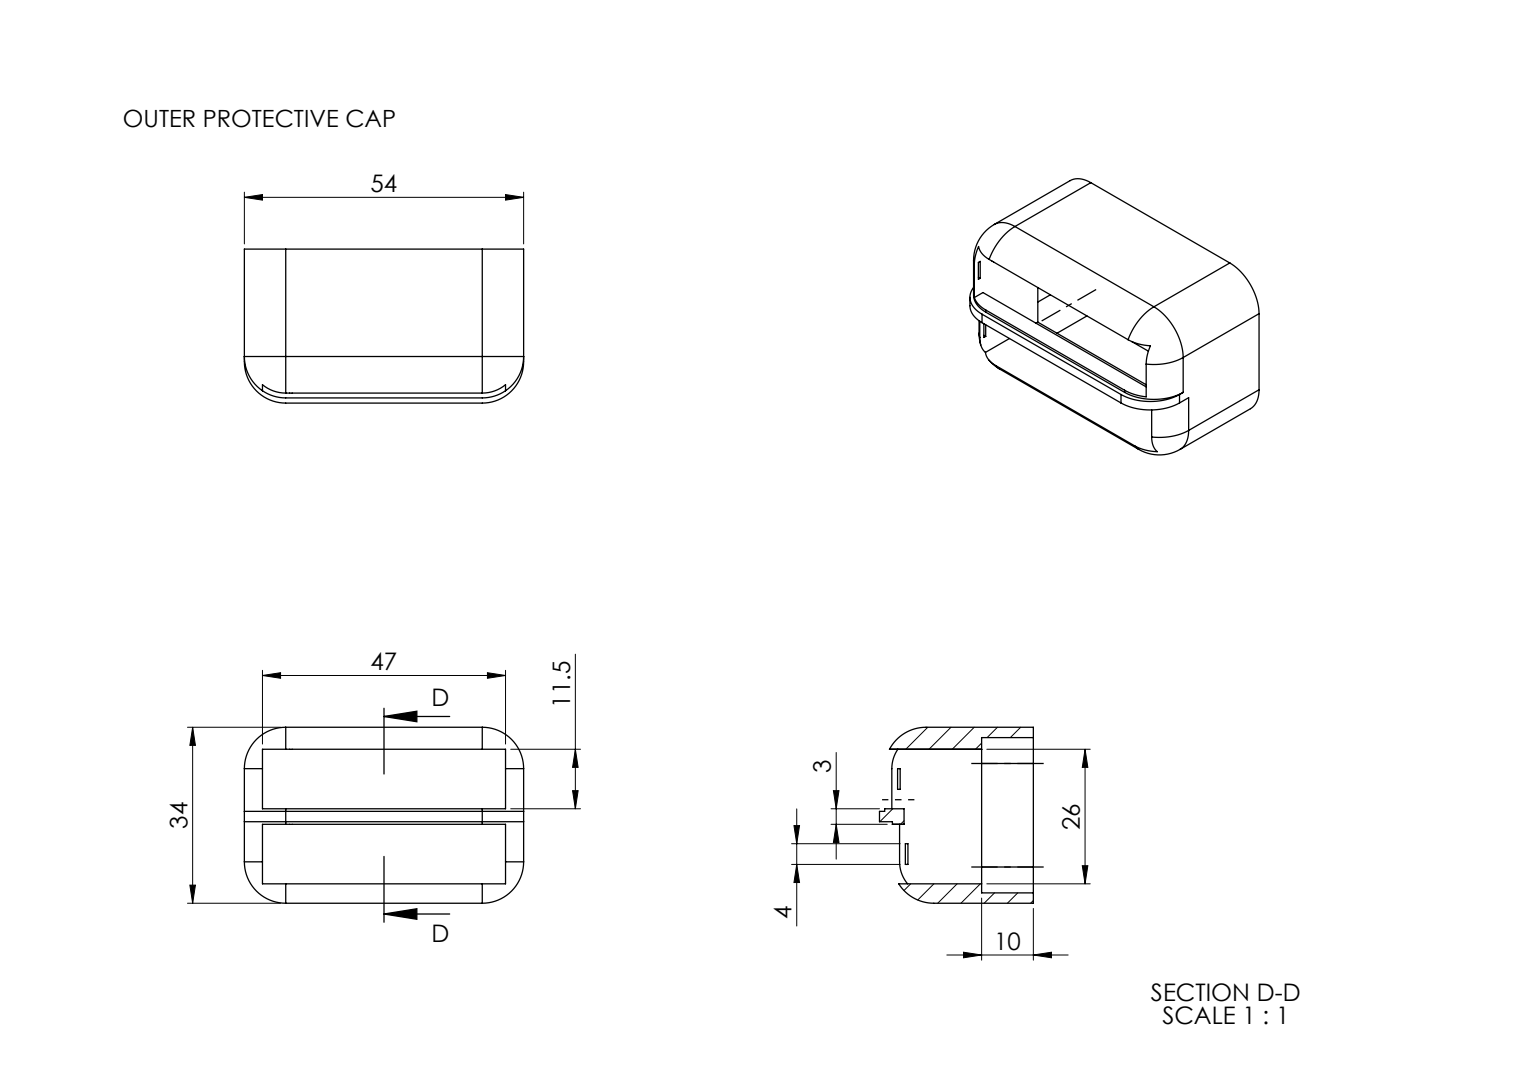
ISO-10303-21;
HEADER;
FILE_DESCRIPTION (('STEP AP214'),
    '1' );
FILE_NAME ('Outer Protective Cap.step',
    '2026-10-05T05:16:24',
    ( '' ),
    ( '' ),
    'SwSTEP 2.0',
    'SolidWorks 2026',
    '' );
FILE_SCHEMA (( 'AUTOMOTIVE_DESIGN' ));
ENDSEC;

DATA;
#39=VERTEX_POINT ( 'NONE', #74855 ) ;
#111=EDGE_LOOP ( 'NONE', ( #30455, #63884, #82521, #35885, #30536 ) ) ;
#125=ORIENTED_EDGE ( 'NONE', *, *, #59924, .F. ) ;
#176=DIRECTION ( 'NONE',  ( -1.000000000000000000, 1.799314243699348838E-16, 0.000000000000000000 ) ) ;
#177=VERTEX_POINT ( 'NONE', #56344 ) ;
#218=CYLINDRICAL_SURFACE ( 'NONE', #17781, 4.999999999999997335 ) ;
#355=CARTESIAN_POINT ( 'NONE',  ( -19.00000000000000355, 12.75000000000000888, 23.75000000000000000 ) ) ;
#369=EDGE_CURVE ( 'NONE', #87698, #17125, #35522, .T. ) ;
#423=VERTEX_POINT ( 'NONE', #22006 ) ;
#439=ORIENTED_EDGE ( 'NONE', *, *, #3601, .F. ) ;
#451=ORIENTED_EDGE ( 'NONE', *, *, #81392, .T. ) ;
#483=DIRECTION ( 'NONE',  ( -1.845450506358306311E-16, 1.000000000000000000, -5.102127870520021228E-17 ) ) ;
#523=VECTOR ( 'NONE', #26290, 1000.000000000000000 ) ;
#545=VERTEX_POINT ( 'NONE', #25105 ) ;
#584=DIRECTION ( 'NONE',  ( -1.000000000000000000, -0.000000000000000000, 0.000000000000000000 ) ) ;
#617=AXIS2_PLACEMENT_3D ( 'NONE', #45736, #44381, #25020 ) ;
#659=ORIENTED_EDGE ( 'NONE', *, *, #57921, .F. ) ;
#717=ADVANCED_FACE ( 'NONE', ( #61106 ), #88613, .F. ) ;
#728=DIRECTION ( 'NONE',  ( -1.000000000000000000, -0.000000000000000000, -0.000000000000000000 ) ) ;
#753=ORIENTED_EDGE ( 'NONE', *, *, #12775, .F. ) ;
#801=DIRECTION ( 'NONE',  ( -0.000000000000000000, -0.000000000000000000, -1.000000000000000000 ) ) ;
#834=DIRECTION ( 'NONE',  ( 0.000000000000000000, -1.000000000000000000, -0.000000000000000000 ) ) ;
#841=LINE ( 'NONE', #21553, #59983 ) ;
#876=ORIENTED_EDGE ( 'NONE', *, *, #18715, .F. ) ;
#913=CARTESIAN_POINT ( 'NONE',  ( 19.99999999999997513, -14.99999999999999467, 3.000000000000000888 ) ) ;
#976=CARTESIAN_POINT ( 'NONE',  ( -24.00000000000000000, 5.000000000000023093, 29.24999999999999645 ) ) ;
#1023=CIRCLE ( 'NONE', #35556, 4.755951259987792668 ) ;
#1024=DIRECTION ( 'NONE',  ( -0.000000000000000000, -0.000000000000000000, -1.000000000000000000 ) ) ;
#1050=CARTESIAN_POINT ( 'NONE',  ( 23.49999999999999645, 1.250000000000003775, 28.00000000000000000 ) ) ;
#1086=EDGE_CURVE ( 'NONE', #31481, #54731, #6721, .T. ) ;
#1098=DIRECTION ( 'NONE',  ( 0.000000000000000000, -1.084202172485503448E-16, 1.000000000000000000 ) ) ;
#1117=ORIENTED_EDGE ( 'NONE', *, *, #87020, .T. ) ;
#1198=CARTESIAN_POINT ( 'NONE',  ( 23.49999999999998934, 12.75000000000000711, 13.00000000000000178 ) ) ;
#1213=EDGE_LOOP ( 'NONE', ( #27297, #63065, #59456, #32063, #63736, #10968 ) ) ;
#1230=CARTESIAN_POINT ( 'NONE',  ( 20.00000000000000711, -9.999999999999994671, 13.00000000000000178 ) ) ;
#1264=DIRECTION ( 'NONE',  ( 0.000000000000000000, 8.131516293641283255E-17, 1.000000000000000000 ) ) ;
#1305=DIRECTION ( 'NONE',  ( 0.000000000000000000, -1.835858764360062270E-15, -1.000000000000000000 ) ) ;
#1341=EDGE_CURVE ( 'NONE', #39, #63016, #10830, .T. ) ;
#1369=VERTEX_POINT ( 'NONE', #40966 ) ;
#1370=DIRECTION ( 'NONE',  ( -8.673617379884044347E-16, 1.000000000000000000, -5.102127870520020612E-17 ) ) ;
#1444=CARTESIAN_POINT ( 'NONE',  ( 19.00000000000000000, 1.250000000000002220, 23.75000000000000000 ) ) ;
#1480=CARTESIAN_POINT ( 'NONE',  ( -17.76215049426127024, 12.75000000000001599, 30.81664701255127881 ) ) ;
#1523=DIRECTION ( 'NONE',  ( -1.000000000000000000, 5.997714145664496128E-17, -5.202187765341190574E-33 ) ) ;
#1557=LINE ( 'NONE', #29045, #38017 ) ;
#1675=VERTEX_POINT ( 'NONE', #16580 ) ;
#1704=FACE_OUTER_BOUND ( 'NONE', #66995, .T. ) ;
#2006=EDGE_CURVE ( 'NONE', #35616, #13977, #81696, .T. ) ;
#2165=CARTESIAN_POINT ( 'NONE',  ( 24.00000000000000000, 9.000000000000024869, 28.74999999999999645 ) ) ;
#2179=FILL_AREA_STYLE ('',( #15712 ) ) ;
#2260=ORIENTED_EDGE ( 'NONE', *, *, #66486, .F. ) ;
#2280=DIRECTION ( 'NONE',  ( -0.000000000000000000, -5.102127870520021228E-17, -1.000000000000000000 ) ) ;
#2292=CARTESIAN_POINT ( 'NONE',  ( 27.00000000000000000, 1.250000000000004663, 31.75000000000000000 ) ) ;
#2302=CARTESIAN_POINT ( 'NONE',  ( 19.00000000000000000, 17.00000000000000000, 2.999999999999999112 ) ) ;
#2374=CARTESIAN_POINT ( 'NONE',  ( -19.99999999999996803, 15.00000000000000711, 3.000000000000000000 ) ) ;
#2474=EDGE_CURVE ( 'NONE', #45845, #16480, #75885, .T. ) ;
#2476=CIRCLE ( 'NONE', #28394, 7.066647012551277918 ) ;
#2479=VERTEX_POINT ( 'NONE', #79605 ) ;
#2506=EDGE_LOOP ( 'NONE', ( #86542, #44118, #22143, #15946, #48903, #37980, #41332, #20143 ) ) ;
#2517=CARTESIAN_POINT ( 'NONE',  ( 27.00000000000000355, -1.749999999999999778, 30.25000000000000000 ) ) ;
#2532=ORIENTED_EDGE ( 'NONE', *, *, #18031, .T. ) ;
#2573=EDGE_CURVE ( 'NONE', #6905, #67687, #74625, .T. ) ;
#2625=CARTESIAN_POINT ( 'NONE',  ( -19.99999999999996447, -15.00000000000000533, 3.000000000000000000 ) ) ;
#2630=CIRCLE ( 'NONE', #81807, 4.999999999999997335 ) ;
#2700=ORIENTED_EDGE ( 'NONE', *, *, #82394, .F. ) ;
#2732=DIRECTION ( 'NONE',  ( -1.000000000000000000, 5.997714145664496128E-17, 0.000000000000000000 ) ) ;
#2785=ORIENTED_EDGE ( 'NONE', *, *, #6461, .T. ) ;
#2797=CARTESIAN_POINT ( 'NONE',  ( -19.99999999999996803, 15.00000000000000711, 13.00000000000000178 ) ) ;
#2836=LINE ( 'NONE', #37071, #56430 ) ;
#2885=VERTEX_POINT ( 'NONE', #13586 ) ;
#2953=VECTOR ( 'NONE', #7163, 1000.000000000000000 ) ;
#3016=CIRCLE ( 'NONE', #41878, 8.000000000000000000 ) ;
#3057=VERTEX_POINT ( 'NONE', #58111 ) ;
#3136=FACE_OUTER_BOUND ( 'NONE', #20499, .T. ) ;
#3200=ORIENTED_EDGE ( 'NONE', *, *, #34878, .F. ) ;
#3233=CARTESIAN_POINT ( 'NONE',  ( -23.50000000000000000, 9.000000000000024869, 28.74999999999999645 ) ) ;
#3297=SPHERICAL_SURFACE ( 'NONE', #10520, 8.000000000000000000 ) ;
#3359=CARTESIAN_POINT ( 'NONE',  ( 27.00000000000000000, 8.999999999999996447, 23.75000000000000000 ) ) ;
#3372=LINE ( 'NONE', #72275, #49878 ) ;
#3387=DIRECTION ( 'NONE',  ( 0.000000000000000000, -2.546383084002652634E-16, -1.000000000000000000 ) ) ;
#3399=ORIENTED_EDGE ( 'NONE', *, *, #32573, .T. ) ;
#3419=COLOUR_RGB ( '', 0.09019608, 0.27058824, 0.51372549) ;
#3420=VECTOR ( 'NONE', #31207, 1000.000000000000000 ) ;
#3466=EDGE_LOOP ( 'NONE', ( #67477, #25046, #38237, #39668, #79080, #56446 ) ) ;
#3504=( NAMED_UNIT ( * ) SI_UNIT ( $, .STERADIAN. ) SOLID_ANGLE_UNIT ( ) );
#3518=EDGE_CURVE ( 'NONE', #44526, #16365, #12061, .T. ) ;
#3601=EDGE_CURVE ( 'NONE', #21923, #31481, #62869, .T. ) ;
#3614=VECTOR ( 'NONE', #80699, 1000.000000000000000 ) ;
#3635=ORIENTED_EDGE ( 'NONE', *, *, #64166, .F. ) ;
#3658=ORIENTED_EDGE ( 'NONE', *, *, #34878, .T. ) ;
#3688=VERTEX_POINT ( 'NONE', #56578 ) ;
#3726=VERTEX_POINT ( 'NONE', #29556 ) ;
#3740=PLANE ( 'NONE',  #67370 ) ;
#3752=EDGE_LOOP ( 'NONE', ( #12490, #71544, #35024, #451, #52192 ) ) ;
#3764=VECTOR ( 'NONE', #64961, 1000.000000000000000 ) ;
#3860=DIRECTION ( 'NONE',  ( 0.000000000000000000, -8.673617379884028076E-17, -1.000000000000000000 ) ) ;
#3878=ORIENTED_EDGE ( 'NONE', *, *, #69519, .F. ) ;
#3888=FACE_OUTER_BOUND ( 'NONE', #46997, .T. ) ;
#3928=VECTOR ( 'NONE', #10062, 1000.000000000000000 ) ;
#3948=ORIENTED_EDGE ( 'NONE', *, *, #34547, .F. ) ;
#3952=VECTOR ( 'NONE', #74260, 1000.000000000000000 ) ;
#3976=ORIENTED_EDGE ( 'NONE', *, *, #4874, .T. ) ;
#4003=CARTESIAN_POINT ( 'NONE',  ( 19.99999999999996803, 15.00000000000000711, 3.000000000000000000 ) ) ;
#4012=AXIS2_PLACEMENT_3D ( 'NONE', #47900, #19109, #88476 ) ;
#4025=CARTESIAN_POINT ( 'NONE',  ( -24.00000000000000000, 5.000000000000023093, 28.74999999999999645 ) ) ;
#4098=CARTESIAN_POINT ( 'NONE',  ( 19.00000000000000000, -13.24999999999999822, 22.25000000000000000 ) ) ;
#4128=EDGE_CURVE ( 'NONE', #31550, #87883, #51453, .T. ) ;
#4149=VERTEX_POINT ( 'NONE', #66670 ) ;
#4163=DIRECTION ( 'NONE',  ( -1.000000000000000000, -1.734723475976813504E-16, 0.000000000000000000 ) ) ;
#4170=CARTESIAN_POINT ( 'NONE',  ( 23.49999999999998934, -9.499999999999982236, 32.75000000000000000 ) ) ;
#4179=DIRECTION ( 'NONE',  ( 0.000000000000000000, 0.000000000000000000, -1.000000000000000000 ) ) ;
#4246=FACE_OUTER_BOUND ( 'NONE', #51472, .T. ) ;
#4272=CARTESIAN_POINT ( 'NONE',  ( 19.00000000000000000, -9.000000000000001776, 3.000000000000000444 ) ) ;
#4339=VECTOR ( 'NONE', #88764, 1000.000000000000000 ) ;
#4430=VERTEX_POINT ( 'NONE', #52588 ) ;
#4613=AXIS2_PLACEMENT_3D ( 'NONE', #74305, #4163, #7172 ) ;
#4720=EDGE_CURVE ( 'NONE', #43004, #66583, #25016, .T. ) ;
#4766=AXIS2_PLACEMENT_3D ( 'NONE', #70291, #8598, #63525 ) ;
#4874=EDGE_CURVE ( 'NONE', #11165, #85470, #9196, .T. ) ;
#4886=EDGE_LOOP ( 'NONE', ( #16594, #13139, #67745, #50693, #20912, #63814, #12403, #82588, #60363, #32892 ) ) ;
#4972=CARTESIAN_POINT ( 'NONE',  ( 19.00000000000000000, 0.7500000000000051070, 32.75000000000000000 ) ) ;
#4981=VECTOR ( 'NONE', #68913, 1000.000000000000000 ) ;
#4993=DIRECTION ( 'NONE',  ( 0.000000000000000000, 0.000000000000000000, -1.000000000000000000 ) ) ;
#5019=DIRECTION ( 'NONE',  ( 0.000000000000000000, 0.000000000000000000, 1.000000000000000000 ) ) ;
#5041=VECTOR ( 'NONE', #66159, 1000.000000000000000 ) ;
#5227=PLANE ( 'NONE',  #65899 ) ;
#5246=CARTESIAN_POINT ( 'NONE',  ( -20.00000000000000355, -10.00000000000000533, 3.000000000000000000 ) ) ;
#5314=ORIENTED_EDGE ( 'NONE', *, *, #30408, .T. ) ;
#5316=EDGE_CURVE ( 'NONE', #76174, #11728, #59705, .T. ) ;
#5331=AXIS2_PLACEMENT_3D ( 'NONE', #20450, #41165, #176 ) ;
#5342=ADVANCED_FACE ( 'NONE', ( #24133 ), #71881, .F. ) ;
#5357=DIRECTION ( 'NONE',  ( -1.000000000000000000, 0.000000000000000000, 0.000000000000000000 ) ) ;
#5363=( NAMED_UNIT ( * ) SI_UNIT ( $, .STERADIAN. ) SOLID_ANGLE_UNIT ( ) );
#5367=ORIENTED_EDGE ( 'NONE', *, *, #53165, .F. ) ;
#5421=CARTESIAN_POINT ( 'NONE',  ( 24.00000000000000000, -5.499999999999981348, 27.75000000000000000 ) ) ;
#5486=EDGE_CURVE ( 'NONE', #30238, #88839, #84428, .T. ) ;
#5604=ORIENTED_EDGE ( 'NONE', *, *, #60963, .T. ) ;
#5642=VERTEX_POINT ( 'NONE', #24030 ) ;
#5646=VERTEX_POINT ( 'NONE', #59598 ) ;
#5699=ORIENTED_EDGE ( 'NONE', *, *, #76759, .F. ) ;
#5731=CARTESIAN_POINT ( 'NONE',  ( -23.50000000000000000, -4.999999999999999112, 28.00000000000000000 ) ) ;
#5735=CARTESIAN_POINT ( 'NONE',  ( 19.00000000000000000, -8.999999999999996447, 22.25000000000000000 ) ) ;
#5821=CARTESIAN_POINT ( 'NONE',  ( 23.49999999999998934, 1.674711738930281374E-15, 32.75000000000000000 ) ) ;
#5872=DIRECTION ( 'NONE',  ( 0.000000000000000000, 1.000000000000000000, 0.000000000000000000 ) ) ;
#5905=CYLINDRICAL_SURFACE ( 'NONE', #8415, 8.000000000000000000 ) ;
#5934=AXIS2_PLACEMENT_3D ( 'NONE', #51338, #37863, #45051 ) ;
#5952=LINE ( 'NONE', #26658, #24339 ) ;
#6010=VERTEX_POINT ( 'NONE', #26600 ) ;
#6014=CARTESIAN_POINT ( 'NONE',  ( 27.00000000000000000, -1.249999999999999112, 32.75000000000000000 ) ) ;
#6025=CARTESIAN_POINT ( 'NONE',  ( -24.00000000000000000, 9.000000000000024869, 29.25000000000000000 ) ) ;
#6048=CARTESIAN_POINT ( 'NONE',  ( 27.00000000000000000, -9.000000000000001776, 2.291744775602387568E-15 ) ) ;
#6069=CIRCLE ( 'NONE', #42074, 8.000000000000000000 ) ;
#6212=VECTOR ( 'NONE', #16061, 1000.000000000000000 ) ;
#6245=VECTOR ( 'NONE', #1098, 1000.000000000000000 ) ;
#6323=ADVANCED_FACE ( 'NONE', ( #53961 ), #81453, .T. ) ;
#6341=VECTOR ( 'NONE', #57691, 1000.000000000000000 ) ;
#6419=DIRECTION ( 'NONE',  ( -1.000000000000000000, 0.000000000000000000, 0.000000000000000000 ) ) ;
#6428=EDGE_CURVE ( 'NONE', #1675, #87698, #55728, .T. ) ;
#6459=ORIENTED_EDGE ( 'NONE', *, *, #78541, .F. ) ;
#6461=EDGE_CURVE ( 'NONE', #24326, #60483, #18351, .T. ) ;
#6465=ORIENTED_EDGE ( 'NONE', *, *, #8401, .F. ) ;
#6483=CYLINDRICAL_SURFACE ( 'NONE', #4012, 4.755951259987790891 ) ;
#6495=PLANE ( 'NONE',  #5331 ) ;
#6503=CIRCLE ( 'NONE', #79853, 8.000000000000000000 ) ;
#6589=ORIENTED_EDGE ( 'NONE', *, *, #17057, .F. ) ;
#6714=LINE ( 'NONE', #48575, #2953 ) ;
#6721=CIRCLE ( 'NONE', #57038, 7.066647012551277918 ) ;
#6795=ADVANCED_FACE ( 'NONE', ( #39027, #31822 ), #5227, .F. ) ;
#6808=DIRECTION ( 'NONE',  ( -1.000000000000000000, 0.000000000000000000, 0.000000000000000000 ) ) ;
#6905=VERTEX_POINT ( 'NONE', #78005 ) ;
#6909=ORIENTED_EDGE ( 'NONE', *, *, #29491, .T. ) ;
#6949=EDGE_LOOP ( 'NONE', ( #61040, #37601, #63641, #78757, #20835, #88190, #51917, #53034, #28989, #28438 ) ) ;
#6996=VECTOR ( 'NONE', #75423, 1000.000000000000000 ) ;
#7127=CARTESIAN_POINT ( 'NONE',  ( -19.99999999999996803, 15.00000000000000711, 13.00000000000000178 ) ) ;
#7136=DIRECTION ( 'NONE',  ( 0.000000000000000000, 1.000000000000000000, 8.673617379884033500E-16 ) ) ;
#7163=DIRECTION ( 'NONE',  ( -0.000000000000000000, -5.102127870520021228E-17, -1.000000000000000000 ) ) ;
#7172=DIRECTION ( 'NONE',  ( 1.734723475976813504E-16, -1.000000000000000000, 0.000000000000000000 ) ) ;
#7189=LINE ( 'NONE', #27018, #85069 ) ;
#7271=DIRECTION ( 'NONE',  ( 0.000000000000000000, 0.000000000000000000, 1.000000000000000000 ) ) ;
#7286=EDGE_LOOP ( 'NONE', ( #59348, #15601, #28024, #83746 ) ) ;
#7302=VECTOR ( 'NONE', #32279, 1000.000000000000000 ) ;
#7321=EDGE_CURVE ( 'NONE', #76030, #46479, #65704, .T. ) ;
#7424=PRODUCT ( 'Outer Protective Cap', 'Outer Protective Cap', '', ( #53651 ) ) ;
#7435=EDGE_CURVE ( 'NONE', #79431, #62505, #2630, .T. ) ;
#7437=EDGE_LOOP ( 'NONE', ( #68832, #81407, #41481, #25142 ) ) ;
#7496=CARTESIAN_POINT ( 'NONE',  ( -23.50000000000000000, 12.75000000000000533, 32.75000000000000000 ) ) ;
#7508=PLANE ( 'NONE',  #35416 ) ;
#7555=DIRECTION ( 'NONE',  ( -1.000000000000000000, -9.819216796286635314E-16, -2.454804199071659026E-15 ) ) ;
#7556=DIRECTION ( 'NONE',  ( 1.000000000000000000, 0.000000000000000000, 0.000000000000000000 ) ) ;
#7579=PRESENTATION_STYLE_ASSIGNMENT (( #34156 ) ) ;
#7587=CARTESIAN_POINT ( 'NONE',  ( -24.00000000000000000, -9.499999999999982236, 27.74999999999999645 ) ) ;
#7626=VERTEX_POINT ( 'NONE', #72360 ) ;
#7648=CARTESIAN_POINT ( 'NONE',  ( -24.00000000000000000, 9.000000000000024869, 28.74999999999999645 ) ) ;
#7726=CARTESIAN_POINT ( 'NONE',  ( 23.49999999999998934, -9.499999999999982236, 27.24999999999999645 ) ) ;
#7740=EDGE_LOOP ( 'NONE', ( #55686, #47275, #8190, #46826, #38658, #51031, #61137, #86767 ) ) ;
#7762=DIRECTION ( 'NONE',  ( 5.997714145664496128E-17, 1.000000000000000000, -5.102127870520021228E-17 ) ) ;
#7817=VERTEX_POINT ( 'NONE', #53418 ) ;
#7988=DIRECTION ( 'NONE',  ( -1.000000000000000000, 1.681660752236433198E-16, 0.000000000000000000 ) ) ;
#8011=DIRECTION ( 'NONE',  ( 0.000000000000000000, -1.000000000000000000, 0.000000000000000000 ) ) ;
#8013=VERTEX_POINT ( 'NONE', #57860 ) ;
#8034=CARTESIAN_POINT ( 'NONE',  ( -19.00000000000000000, -1.249999999999997558, 22.25000000000000000 ) ) ;
#8098=ORIENTED_EDGE ( 'NONE', *, *, #38884, .T. ) ;
#8113=ORIENTED_EDGE ( 'NONE', *, *, #2474, .T. ) ;
#8128=LINE ( 'NONE', #8570, #54588 ) ;
#8138=PLANE ( 'NONE',  #17965 ) ;
#8140=CARTESIAN_POINT ( 'NONE',  ( -17.76215049426128445, -1.749999999999992450, 28.00000000000000000 ) ) ;
#8190=ORIENTED_EDGE ( 'NONE', *, *, #7435, .F. ) ;
#8196=CARTESIAN_POINT ( 'NONE',  ( 23.49999999999999645, -4.999999999999999112, 28.00000000000000000 ) ) ;
#8219=VERTEX_POINT ( 'NONE', #1050 ) ;
#8232=DIRECTION ( 'NONE',  ( 0.000000000000000000, 0.000000000000000000, -1.000000000000000000 ) ) ;
#8240=CARTESIAN_POINT ( 'NONE',  ( 24.00000000000000000, 5.000000000000023093, 29.24999999999999645 ) ) ;
#8260=VECTOR ( 'NONE', #9877, 1000.000000000000000 ) ;
#8266=ORIENTED_EDGE ( 'NONE', *, *, #26687, .F. ) ;
#8267=VECTOR ( 'NONE', #45746, 1000.000000000000000 ) ;
#8384=DIRECTION ( 'NONE',  ( 0.000000000000000000, 0.000000000000000000, -1.000000000000000000 ) ) ;
#8401=EDGE_CURVE ( 'NONE', #11121, #17125, #86987, .T. ) ;
#8415=AXIS2_PLACEMENT_3D ( 'NONE', #33381, #60839, #33813 ) ;
#8570=CARTESIAN_POINT ( 'NONE',  ( 23.49999999999998579, -13.25000000000000000, 32.75000000000000000 ) ) ;
#8590=DIRECTION ( 'NONE',  ( -1.000000000000000000, 0.000000000000000000, -0.000000000000000000 ) ) ;
#8598=DIRECTION ( 'NONE',  ( 0.000000000000000000, -5.102127870520020612E-17, -1.000000000000000000 ) ) ;
#8626=LINE ( 'NONE', #36535, #16851 ) ;
#8636=LINE ( 'NONE', #2292, #13220 ) ;
#8670=DIRECTION ( 'NONE',  ( 0.000000000000000000, 1.084202172485504434E-16, -1.000000000000000000 ) ) ;
#8720=DIRECTION ( 'NONE',  ( -0.000000000000000000, 1.000000000000000000, 0.000000000000000000 ) ) ;
#8746=ADVANCED_FACE ( 'NONE', ( #30164 ), #49552, .F. ) ;
#8750=EDGE_CURVE ( 'NONE', #87698, #26806, #49101, .T. ) ;
#8767=DIRECTION ( 'NONE',  ( 0.000000000000000000, -1.000000000000000000, 0.000000000000000000 ) ) ;
#8791=DIRECTION ( 'NONE',  ( -0.000000000000000000, -1.000000000000000000, -8.673617379884033500E-16 ) ) ;
#8793=AXIS2_PLACEMENT_3D ( 'NONE', #28742, #56206, #42260 ) ;
#8833=CARTESIAN_POINT ( 'NONE',  ( -27.00000000000000000, 0.7500000000000059952, 24.75000000000000000 ) ) ;
#8844=EDGE_CURVE ( 'NONE', #79547, #52311, #8128, .T. ) ;
#8863=ORIENTED_EDGE ( 'NONE', *, *, #8401, .T. ) ;
#8892=ORIENTED_EDGE ( 'NONE', *, *, #22887, .F. ) ;
#9065=EDGE_LOOP ( 'NONE', ( #69141, #36454, #49626, #49654 ) ) ;
#9076=AXIS2_PLACEMENT_3D ( 'NONE', #58222, #44698, #23116 ) ;
#9108=ORIENTED_EDGE ( 'NONE', *, *, #84957, .T. ) ;
#9143=ORIENTED_EDGE ( 'NONE', *, *, #25495, .T. ) ;
#9196=LINE ( 'NONE', #71314, #3928 ) ;
#9238=CARTESIAN_POINT ( 'NONE',  ( -24.00000000000000000, 9.000000000000024869, 29.25000000000000000 ) ) ;
#9245=ADVANCED_FACE ( 'NONE', ( #4246 ), #32605, .F. ) ;
#9328=EDGE_LOOP ( 'NONE', ( #60045, #3948, #71017, #78144 ) ) ;
#9390=ORIENTED_EDGE ( 'NONE', *, *, #12535, .F. ) ;
#9391=LINE ( 'NONE', #44479, #86633 ) ;
#9442=DIRECTION ( 'NONE',  ( -0.000000000000000000, -0.000000000000000000, -1.000000000000000000 ) ) ;
#9446=DIRECTION ( 'NONE',  ( 0.000000000000000000, 0.000000000000000000, 1.000000000000000000 ) ) ;
#9454=EDGE_CURVE ( 'NONE', #81222, #85470, #45970, .T. ) ;
#9506=ORIENTED_EDGE ( 'NONE', *, *, #18954, .T. ) ;
#9638=ORIENTED_EDGE ( 'NONE', *, *, #38910, .T. ) ;
#9679=EDGE_CURVE ( 'NONE', #76954, #66225, #76195, .T. ) ;
#9687=ORIENTED_EDGE ( 'NONE', *, *, #70774, .F. ) ;
#9877=DIRECTION ( 'NONE',  ( -0.000000000000000000, -0.000000000000000000, -1.000000000000000000 ) ) ;
#9880=DIRECTION ( 'NONE',  ( 1.000000000000000000, -0.000000000000000000, -0.000000000000000000 ) ) ;
#9914=ORIENTED_EDGE ( 'NONE', *, *, #12070, .F. ) ;
#9922=VERTEX_POINT ( 'NONE', #15788 ) ;
#9924=FACE_OUTER_BOUND ( 'NONE', #12091, .T. ) ;
#10003=ORIENTED_EDGE ( 'NONE', *, *, #60963, .F. ) ;
#10009=LINE ( 'NONE', #2797, #85627 ) ;
#10062=DIRECTION ( 'NONE',  ( -0.000000000000000000, 1.000000000000000000, -0.000000000000000000 ) ) ;
#10068=VECTOR ( 'NONE', #29097, 1000.000000000000000 ) ;
#10078=DIRECTION ( 'NONE',  ( -0.000000000000000000, 1.000000000000000000, -0.000000000000000000 ) ) ;
#10191=CARTESIAN_POINT ( 'NONE',  ( -24.00000000000000000, -5.499999999999981348, 27.75000000000000000 ) ) ;
#10198=AXIS2_PLACEMENT_3D ( 'NONE', #51631, #79136, #17437 ) ;
#10253=DIRECTION ( 'NONE',  ( 0.000000000000000000, -1.000000000000000000, -8.673617379884033500E-16 ) ) ;
#10353=CARTESIAN_POINT ( 'NONE',  ( 27.00000000000000000, -16.99999999999999289, 30.25000000000000000 ) ) ;
#10520=AXIS2_PLACEMENT_3D ( 'NONE', #59132, #37525, #64991 ) ;
#10602=CARTESIAN_POINT ( 'NONE',  ( 23.49999999999998934, 12.75000000000000888, 32.75000000000000000 ) ) ;
#10661=PLANE ( 'NONE',  #23127 ) ;
#10666=DIRECTION ( 'NONE',  ( 0.000000000000000000, 0.000000000000000000, -1.000000000000000000 ) ) ;
#10732=VECTOR ( 'NONE', #79377, 1000.000000000000000 ) ;
#10742=ORIENTED_EDGE ( 'NONE', *, *, #73680, .F. ) ;
#10782=LINE ( 'NONE', #30165, #5041 ) ;
#10819=PLANE ( 'NONE',  #74194 ) ;
#10830=LINE ( 'NONE', #80639, #41309 ) ;
#10912=LINE ( 'NONE', #70848, #72096 ) ;
#10943=ORIENTED_EDGE ( 'NONE', *, *, #30776, .F. ) ;
#10968=ORIENTED_EDGE ( 'NONE', *, *, #71445, .F. ) ;
#11027=DIRECTION ( 'NONE',  ( -0.000000000000000000, -5.102127870520021228E-17, -1.000000000000000000 ) ) ;
#11028=ORIENTED_EDGE ( 'NONE', *, *, #20816, .T. ) ;
#11082=EDGE_CURVE ( 'NONE', #65772, #45114, #6714, .T. ) ;
#11121=VERTEX_POINT ( 'NONE', #55339 ) ;
#11142=AXIS2_PLACEMENT_3D ( 'NONE', #10191, #52495, #66467 ) ;
#11165=VERTEX_POINT ( 'NONE', #60771 ) ;
#11270=CARTESIAN_POINT ( 'NONE',  ( 24.00000000000000000, 9.000000000000024869, 29.25000000000000000 ) ) ;
#11394=DIRECTION ( 'NONE',  ( -1.000000000000000000, 0.000000000000000000, 0.000000000000000000 ) ) ;
#11416=VECTOR ( 'NONE', #32266, 1000.000000000000000 ) ;
#11440=CARTESIAN_POINT ( 'NONE',  ( 23.49999999999998934, -9.499999999999982236, 27.74999999999999645 ) ) ;
#11472=LINE ( 'NONE', #79929, #40463 ) ;
#11479=CARTESIAN_POINT ( 'NONE',  ( -23.50000000000000000, 1.250000000000005329, 32.75000000000000000 ) ) ;
#11544=CARTESIAN_POINT ( 'NONE',  ( 27.00000000000000000, 17.00000000000000000, 2.999999999999999112 ) ) ;
#11580=DIRECTION ( 'NONE',  ( 1.000000000000000000, -0.000000000000000000, -0.000000000000000000 ) ) ;
#11610=DIRECTION ( 'NONE',  ( 0.000000000000000000, 1.000000000000000000, -8.673617379884035472E-17 ) ) ;
#11625=PRODUCT_DEFINITION_FORMATION_WITH_SPECIFIED_SOURCE ( 'ANY', '', #7424, .NOT_KNOWN. ) ;
#11661=DIRECTION ( 'NONE',  ( 0.000000000000000000, -1.000000000000000000, 4.336808689942017736E-16 ) ) ;
#11684=ORIENTED_EDGE ( 'NONE', *, *, #44990, .F. ) ;
#11728=VERTEX_POINT ( 'NONE', #55960 ) ;
#11777=ORIENTED_EDGE ( 'NONE', *, *, #68590, .T. ) ;
#11801=ORIENTED_EDGE ( 'NONE', *, *, #55924, .T. ) ;
#11815=DIRECTION ( 'NONE',  ( 0.000000000000000000, -1.734723475976807094E-15, 1.000000000000000000 ) ) ;
#11898=CARTESIAN_POINT ( 'NONE',  ( -24.00000000000000000, -5.499999999999981348, 27.25000000000000000 ) ) ;
#11968=EDGE_CURVE ( 'NONE', #58506, #69466, #3016, .T. ) ;
#12061=LINE ( 'NONE', #5731, #21237 ) ;
#12070=EDGE_CURVE ( 'NONE', #64945, #68629, #11472, .T. ) ;
#12091=EDGE_LOOP ( 'NONE', ( #9390, #73108, #41023, #25285 ) ) ;
#12093=EDGE_LOOP ( 'NONE', ( #35540, #62139, #69676, #3635 ) ) ;
#12118=CARTESIAN_POINT ( 'NONE',  ( 27.00000000000000000, 16.99999999999999289, 31.75000000000000000 ) ) ;
#12132=EDGE_LOOP ( 'NONE', ( #40428, #59501, #85620, #21590 ) ) ;
#12133=AXIS2_PLACEMENT_3D ( 'NONE', #47495, #34430, #34866 ) ;
#12180=CIRCLE ( 'NONE', #20789, 7.999999999999998224 ) ;
#12194=FACE_OUTER_BOUND ( 'NONE', #55388, .T. ) ;
#12341=AXIS2_PLACEMENT_3D ( 'NONE', #80947, #39070, #65182 ) ;
#12400=DIRECTION ( 'NONE',  ( -0.000000000000000000, -5.102127870520021228E-17, -1.000000000000000000 ) ) ;
#12403=ORIENTED_EDGE ( 'NONE', *, *, #79194, .F. ) ;
#12427=CARTESIAN_POINT ( 'NONE',  ( 19.00000000000000000, -17.00000000000000000, 2.999999999999999112 ) ) ;
#12478=AXIS2_PLACEMENT_3D ( 'NONE', #7587, #47680, #14337 ) ;
#12490=ORIENTED_EDGE ( 'NONE', *, *, #75862, .F. ) ;
#12528=ORIENTED_EDGE ( 'NONE', *, *, #57921, .T. ) ;
#12529=EDGE_CURVE ( 'NONE', #43877, #88176, #27980, .T. ) ;
#12535=EDGE_CURVE ( 'NONE', #31022, #56583, #72080, .T. ) ;
#12737=ORIENTED_EDGE ( 'NONE', *, *, #80670, .F. ) ;
#12775=EDGE_CURVE ( 'NONE', #13977, #73914, #87377, .T. ) ;
#12832=ORIENTED_EDGE ( 'NONE', *, *, #60564, .T. ) ;
#12961=EDGE_CURVE ( 'NONE', #47159, #43004, #52013, .T. ) ;
#13110=DIRECTION ( 'NONE',  ( 0.000000000000000000, 1.000000000000000000, 0.000000000000000000 ) ) ;
#13139=ORIENTED_EDGE ( 'NONE', *, *, #87746, .T. ) ;
#13141=DIRECTION ( 'NONE',  ( 1.000000000000000000, 0.000000000000000000, 0.000000000000000000 ) ) ;
#13181=ADVANCED_FACE ( 'NONE', ( #88945 ), #55126, .T. ) ;
#13220=VECTOR ( 'NONE', #2732, 1000.000000000000000 ) ;
#13419=CARTESIAN_POINT ( 'NONE',  ( -39.05038313613820122, 12.25000000000000711, 28.74999999999999645 ) ) ;
#13422=DIRECTION ( 'NONE',  ( 0.000000000000000000, -1.000000000000000000, 0.000000000000000000 ) ) ;
#13448=PLANE ( 'NONE',  #12478 ) ;
#13488=CARTESIAN_POINT ( 'NONE',  ( 27.00000000000000000, 0.7500000000000052180, 31.75000000000000000 ) ) ;
#13582=CARTESIAN_POINT ( 'NONE',  ( 23.49999999999998934, 4.710477821889702467E-15, 29.24999999999999289 ) ) ;
#13586=CARTESIAN_POINT ( 'NONE',  ( -19.00000000000000000, 17.00000000000000000, 2.999999999999999112 ) ) ;
#13646=AXIS2_PLACEMENT_3D ( 'NONE', #80003, #19958, #59280 ) ;
#13662=CARTESIAN_POINT ( 'NONE',  ( 25.00000000000000355, 9.999999999999971578, 13.00000000000000178 ) ) ;
#13714=CARTESIAN_POINT ( 'NONE',  ( 27.00000000000000000, 0.000000000000000000, 23.75000000000000000 ) ) ;
#13755=DIRECTION ( 'NONE',  ( 0.000000000000000000, 0.000000000000000000, 1.000000000000000000 ) ) ;
#13820=EDGE_CURVE ( 'NONE', #38892, #11165, #6069, .T. ) ;
#13855=DIRECTION ( 'NONE',  ( -1.000000000000000000, -0.000000000000000000, -0.000000000000000000 ) ) ;
#13869=ORIENTED_EDGE ( 'NONE', *, *, #52559, .F. ) ;
#13883=SURFACE_STYLE_FILL_AREA ( #48105 ) ;
#13920=AXIS2_PLACEMENT_3D ( 'NONE', #60216, #26885, #54343 ) ;
#13977=VERTEX_POINT ( 'NONE', #62544 ) ;
#14033=EDGE_CURVE ( 'NONE', #53401, #77030, #9391, .T. ) ;
#14162=VERTEX_POINT ( 'NONE', #79175 ) ;
#14170=CARTESIAN_POINT ( 'NONE',  ( -20.00000000000000355, -10.00000000000000533, 13.00000000000000178 ) ) ;
#14242=DIRECTION ( 'NONE',  ( 0.000000000000000000, -1.000000000000000000, 0.000000000000000000 ) ) ;
#14284=AXIS2_PLACEMENT_3D ( 'NONE', #71255, #72148, #36602 ) ;
#14294=FACE_OUTER_BOUND ( 'NONE', #9328, .T. ) ;
#14318=CARTESIAN_POINT ( 'NONE',  ( 27.00000000000000000, 0.7500000000000061062, 23.75000000000000000 ) ) ;
#14337=DIRECTION ( 'NONE',  ( 0.000000000000000000, 0.000000000000000000, -1.000000000000000000 ) ) ;
#14379=CIRCLE ( 'NONE', #50288, 4.999999999999997335 ) ;
#14394=ORIENTED_EDGE ( 'NONE', *, *, #79644, .F. ) ;
#14490=EDGE_CURVE ( 'NONE', #62484, #43877, #22349, .T. ) ;
#14577=UNCERTAINTY_MEASURE_WITH_UNIT (LENGTH_MEASURE( 1.000000000000000082E-05 ), #80064, 'distance_accuracy_value', 'NONE');
#14606=LINE ( 'NONE', #13714, #16418 ) ;
#14608=CARTESIAN_POINT ( 'NONE',  ( -25.00000000000000355, 9.999999999999971578, 3.000000000000000000 ) ) ;
#14613=CARTESIAN_POINT ( 'NONE',  ( -18.00000000000001421, 17.49999999999802824, 32.75000000000000000 ) ) ;
#14621=EDGE_LOOP ( 'NONE', ( #8892, #26121, #83182, #81793 ) ) ;
#14656=CARTESIAN_POINT ( 'NONE',  ( -27.00000000000000000, -1.250000000000000000, 22.25000000000000000 ) ) ;
#14706=ORIENTED_EDGE ( 'NONE', *, *, #53045, .F. ) ;
#14716=EDGE_LOOP ( 'NONE', ( #43267, #46097, #3399, #57529 ) ) ;
#14756=CARTESIAN_POINT ( 'NONE',  ( 23.49999999999998934, 5.000000000000023093, 28.74999999999999645 ) ) ;
#14820=ADVANCED_FACE ( 'NONE', ( #71636 ), #57689, .T. ) ;
#14842=AXIS2_PLACEMENT_3D ( 'NONE', #69439, #43300, #55914 ) ;
#14851=DIRECTION ( 'NONE',  ( 0.000000000000000000, -1.000000000000000000, 0.000000000000000000 ) ) ;
#14864=LINE ( 'NONE', #20285, #51703 ) ;
#14890=DIRECTION ( 'NONE',  ( 0.000000000000000000, 0.000000000000000000, -1.000000000000000000 ) ) ;
#14965=ORIENTED_EDGE ( 'NONE', *, *, #28232, .T. ) ;
#14969=ORIENTED_EDGE ( 'NONE', *, *, #56579, .T. ) ;
#15048=LINE ( 'NONE', #42523, #19719 ) ;
#15076=DIRECTION ( 'NONE',  ( 1.000000000000000000, -0.000000000000000000, -0.000000000000000000 ) ) ;
#15105=VECTOR ( 'NONE', #70409, 1000.000000000000000 ) ;
#15156=EDGE_CURVE ( 'NONE', #3726, #58506, #7189, .T. ) ;
#15215=CARTESIAN_POINT ( 'NONE',  ( 19.00000000000000000, 0.000000000000000000, 24.75000000000000000 ) ) ;
#15276=AXIS2_PLACEMENT_3D ( 'NONE', #75743, #6419, #82079 ) ;
#15312=ORIENTED_EDGE ( 'NONE', *, *, #29870, .T. ) ;
#15326=ADVANCED_FACE ( 'NONE', ( #29054 ), #22280, .F. ) ;
#15329=CARTESIAN_POINT ( 'NONE',  ( 24.00000000000000000, 14.50000000000000533, 1.499999999999997780 ) ) ;
#15542=DIRECTION ( 'NONE',  ( -1.799314243699348838E-16, -1.000000000000000000, 5.102127870520021228E-17 ) ) ;
#15585=DIRECTION ( 'NONE',  ( -0.000000000000000000, -5.102127870520021228E-17, -1.000000000000000000 ) ) ;
#15596=CARTESIAN_POINT ( 'NONE',  ( -24.00000000000000000, -9.499999999999982236, 27.74999999999999645 ) ) ;
#15601=ORIENTED_EDGE ( 'NONE', *, *, #84957, .F. ) ;
#15624=EDGE_CURVE ( 'NONE', #44546, #9922, #69323, .T. ) ;
#15654=CARTESIAN_POINT ( 'NONE',  ( 23.49999999999998579, -8.999999999999996447, 28.86437827766148345 ) ) ;
#15712=FILL_AREA_STYLE_COLOUR ( '', #3419 ) ;
#15771=CARTESIAN_POINT ( 'NONE',  ( 24.00000000000000000, 9.000000000000024869, 29.25000000000000000 ) ) ;
#15788=CARTESIAN_POINT ( 'NONE',  ( 27.00000000000000000, 0.7500000000000059952, 24.75000000000000000 ) ) ;
#15849=VERTEX_POINT ( 'NONE', #32928 ) ;
#15943=VERTEX_POINT ( 'NONE', #21176 ) ;
#15946=ORIENTED_EDGE ( 'NONE', *, *, #29149, .T. ) ;
#15976=VECTOR ( 'NONE', #53324, 1000.000000000000000 ) ;
#15985=EDGE_LOOP ( 'NONE', ( #23359, #38033, #42032, #3200 ) ) ;
#15989=LINE ( 'NONE', #9238, #57236 ) ;
#15999=DIRECTION ( 'NONE',  ( 0.000000000000000000, -1.000000000000000000, 4.336808689942017736E-16 ) ) ;
#16061=DIRECTION ( 'NONE',  ( -0.000000000000000000, -0.000000000000000000, -1.000000000000000000 ) ) ;
#16063=ORIENTED_EDGE ( 'NONE', *, *, #42110, .F. ) ;
#16102=CARTESIAN_POINT ( 'NONE',  ( 27.00000000000000000, 0.000000000000000000, 22.25000000000000000 ) ) ;
#16116=EDGE_CURVE ( 'NONE', #56516, #69466, #81019, .T. ) ;
#16138=EDGE_CURVE ( 'NONE', #88830, #56373, #73362, .T. ) ;
#16351=FACE_OUTER_BOUND ( 'NONE', #7286, .T. ) ;
#16365=VERTEX_POINT ( 'NONE', #33495 ) ;
#16418=VECTOR ( 'NONE', #41194, 1000.000000000000000 ) ;
#16427=EDGE_LOOP ( 'NONE', ( #45138, #48937, #69979, #35694 ) ) ;
#16450=ORIENTED_EDGE ( 'NONE', *, *, #50493, .F. ) ;
#16479=AXIS2_PLACEMENT_3D ( 'NONE', #63920, #86445, #37331 ) ;
#16480=VERTEX_POINT ( 'NONE', #83909 ) ;
#16500=DIRECTION ( 'NONE',  ( 0.000000000000000000, -1.000000000000000000, -8.673617379884033500E-16 ) ) ;
#16578=DIRECTION ( 'NONE',  ( 0.000000000000000000, 0.000000000000000000, -1.000000000000000000 ) ) ;
#16580=CARTESIAN_POINT ( 'NONE',  ( 24.00000000000000000, 5.000000000000023093, 28.74999999999999645 ) ) ;
#16594=ORIENTED_EDGE ( 'NONE', *, *, #64615, .T. ) ;
#16731=UNCERTAINTY_MEASURE_WITH_UNIT (LENGTH_MEASURE( 1.000000000000000082E-05 ), #73373, 'distance_accuracy_value', 'NONE');
#16758=CARTESIAN_POINT ( 'NONE',  ( 27.00000000000000000, 0.000000000000000000, 0.000000000000000000 ) ) ;
#16760=CIRCLE ( 'NONE', #52704, 8.000000000000000000 ) ;
#16794=CARTESIAN_POINT ( 'NONE',  ( 7.497142682080633102E-17, 1.250000000000003553, 28.00000000000000000 ) ) ;
#16823=VECTOR ( 'NONE', #23413, 1000.000000000000000 ) ;
#16851=VECTOR ( 'NONE', #2280, 1000.000000000000000 ) ;
#16906=CYLINDRICAL_SURFACE ( 'NONE', #27624, 8.000000000000000000 ) ;
#17055=ORIENTED_EDGE ( 'NONE', *, *, #66336, .T. ) ;
#17057=EDGE_CURVE ( 'NONE', #88830, #13977, #32839, .T. ) ;
#17061=DIRECTION ( 'NONE',  ( 0.000000000000000000, 1.000000000000000000, 8.673617379884034486E-16 ) ) ;
#17081=LINE ( 'NONE', #56739, #8260 ) ;
#17086=AXIS2_PLACEMENT_3D ( 'NONE', #12118, #83229, #54863 ) ;
#17125=VERTEX_POINT ( 'NONE', #33727 ) ;
#17131=EDGE_LOOP ( 'NONE', ( #9506, #70627, #17055, #68156, #39911, #67901, #63783, #41654 ) ) ;
#17294=DIRECTION ( 'NONE',  ( 0.000000000000000000, 0.000000000000000000, 1.000000000000000000 ) ) ;
#17389=VECTOR ( 'NONE', #9880, 1000.000000000000000 ) ;
#17416=LINE ( 'NONE', #80004, #85092 ) ;
#17417=EDGE_LOOP ( 'NONE', ( #2260, #85181, #55144, #53399 ) ) ;
#17437=DIRECTION ( 'NONE',  ( 1.000000000000000000, 0.000000000000000000, 0.000000000000000000 ) ) ;
#17511=LINE ( 'NONE', #51712, #25894 ) ;
#17521=FACE_OUTER_BOUND ( 'NONE', #80523, .T. ) ;
#17591=FACE_OUTER_BOUND ( 'NONE', #38414, .T. ) ;
#17614=ORIENTED_EDGE ( 'NONE', *, *, #33771, .F. ) ;
#17740=ORIENTED_EDGE ( 'NONE', *, *, #73680, .T. ) ;
#17781=AXIS2_PLACEMENT_3D ( 'NONE', #14170, #41646, #69115 ) ;
#17788=ORIENTED_EDGE ( 'NONE', *, *, #50706, .F. ) ;
#17817=DIRECTION ( 'NONE',  ( -0.000000000000000000, -5.102127870520021228E-17, -1.000000000000000000 ) ) ;
#17841=AXIS2_PLACEMENT_3D ( 'NONE', #75858, #75420, #68221 ) ;
#17878=DIRECTION ( 'NONE',  ( 0.000000000000000000, 0.000000000000000000, 1.000000000000000000 ) ) ;
#17925=ORIENTED_EDGE ( 'NONE', *, *, #31578, .F. ) ;
#17965=AXIS2_PLACEMENT_3D ( 'NONE', #83808, #1370, #42374 ) ;
#18018=CARTESIAN_POINT ( 'NONE',  ( 7.497142682080631869E-17, 1.250000000000003775, 32.75000000000000000 ) ) ;
#18031=EDGE_CURVE ( 'NONE', #7626, #2885, #82439, .T. ) ;
#18036=ORIENTED_EDGE ( 'NONE', *, *, #22131, .F. ) ;
#18109=DIRECTION ( 'NONE',  ( 0.000000000000000000, 0.000000000000000000, 1.000000000000000000 ) ) ;
#18122=ORIENTED_EDGE ( 'NONE', *, *, #14490, .T. ) ;
#18127=VECTOR ( 'NONE', #728, 1000.000000000000000 ) ;
#18154=ORIENTED_EDGE ( 'NONE', *, *, #88340, .F. ) ;
#18166=VERTEX_POINT ( 'NONE', #77763 ) ;
#18320=AXIS2_PLACEMENT_3D ( 'NONE', #31184, #34188, #19793 ) ;
#18351=CIRCLE ( 'NONE', #68676, 5.000000000000000888 ) ;
#18359=CARTESIAN_POINT ( 'NONE',  ( -23.50000000000000000, 1.674711738930281374E-15, 13.00000000000000178 ) ) ;
#18380=LINE ( 'NONE', #2625, #49219 ) ;
#18519=CARTESIAN_POINT ( 'NONE',  ( -24.00000000000000000, -9.499999999999982236, 27.74999999999999645 ) ) ;
#18582=EDGE_LOOP ( 'NONE', ( #69344, #44033, #11028, #60832 ) ) ;
#18597=EDGE_CURVE ( 'NONE', #4430, #44526, #27348, .T. ) ;
#18623=CARTESIAN_POINT ( 'NONE',  ( 24.00000000000000000, -5.499999999999981348, 27.25000000000000000 ) ) ;
#18680=EDGE_CURVE ( 'NONE', #52311, #4149, #64658, .T. ) ;
#18715=EDGE_CURVE ( 'NONE', #19020, #34521, #79969, .T. ) ;
#18750=DIRECTION ( 'NONE',  ( -1.000000000000000000, 0.000000000000000000, 0.000000000000000000 ) ) ;
#18755=ORIENTED_EDGE ( 'NONE', *, *, #66486, .T. ) ;
#18863=CARTESIAN_POINT ( 'NONE',  ( 27.00000000000000000, -17.00000000000000000, 2.999999999999999112 ) ) ;
#18905=ADVANCED_FACE ( 'NONE', ( #69114 ), #33994, .T. ) ;
#18953=CARTESIAN_POINT ( 'NONE',  ( 24.00000000000000000, -9.499999999999982236, 27.25000000000000000 ) ) ;
#18954=EDGE_CURVE ( 'NONE', #45845, #9922, #34439, .T. ) ;
#19020=VERTEX_POINT ( 'NONE', #29909 ) ;
#19051=DIRECTION ( 'NONE',  ( 0.000000000000000000, 0.000000000000000000, 1.000000000000000000 ) ) ;
#19098=EDGE_CURVE ( 'NONE', #5646, #2479, #65452, .T. ) ;
#19109=DIRECTION ( 'NONE',  ( -0.000000000000000000, -5.102127870520021228E-17, -1.000000000000000000 ) ) ;
#19122=ORIENTED_EDGE ( 'NONE', *, *, #1086, .F. ) ;
#19125=DIRECTION ( 'NONE',  ( -0.000000000000000000, -5.102127870520021228E-17, -1.000000000000000000 ) ) ;
#19144=ADVANCED_FACE ( 'NONE', ( #79425, #44726 ), #32556, .F. ) ;
#19191=VECTOR ( 'NONE', #17061, 1000.000000000000000 ) ;
#19266=CYLINDRICAL_SURFACE ( 'NONE', #45755, 8.000000000000000000 ) ;
#19307=DIRECTION ( 'NONE',  ( 0.000000000000000000, 1.000000000000000000, 5.102127870520020612E-17 ) ) ;
#19315=AXIS2_PLACEMENT_3D ( 'NONE', #55062, #67255, #27590 ) ;
#19336=FACE_BOUND ( 'NONE', #83331, .T. ) ;
#19352=ORIENTED_EDGE ( 'NONE', *, *, #85635, .F. ) ;
#19360=CARTESIAN_POINT ( 'NONE',  ( -19.00000000000000000, 0.7500000000000041078, 23.75000000000000000 ) ) ;
#19391=DIRECTION ( 'NONE',  ( 1.000000000000000000, 0.000000000000000000, 0.000000000000000000 ) ) ;
#19393=CARTESIAN_POINT ( 'NONE',  ( -24.00000000000000000, -5.499999999999981348, 27.75000000000000000 ) ) ;
#19564=DIRECTION ( 'NONE',  ( 0.000000000000000000, -5.102127870520020612E-17, -1.000000000000000000 ) ) ;
#19625=ADVANCED_FACE ( 'NONE', ( #49518 ), #22043, .T. ) ;
#19643=CARTESIAN_POINT ( 'NONE',  ( -27.00000000000000000, 8.999999999999996447, 23.75000000000000000 ) ) ;
#19703=CARTESIAN_POINT ( 'NONE',  ( -19.00000000000000000, 0.7500000000000051070, 24.75000000000000000 ) ) ;
#19719=VECTOR ( 'NONE', #48819, 1000.000000000000000 ) ;
#19737=DIRECTION ( 'NONE',  ( 1.000000000000000000, 0.000000000000000000, 0.000000000000000000 ) ) ;
#19769=VECTOR ( 'NONE', #76730, 1000.000000000000000 ) ;
#19779=FACE_OUTER_BOUND ( 'NONE', #62503, .T. ) ;
#19793=DIRECTION ( 'NONE',  ( 0.000000000000000000, -1.000000000000000000, 8.673617379884035472E-17 ) ) ;
#19828=LINE ( 'NONE', #43198, #24840 ) ;
#19912=AXIS2_PLACEMENT_3D ( 'NONE', #40103, #68878, #55364 ) ;
#19940=DIRECTION ( 'NONE',  ( 0.000000000000000000, 2.413528314402514090E-16, -1.000000000000000000 ) ) ;
#19958=DIRECTION ( 'NONE',  ( -0.000000000000000000, -0.000000000000000000, -1.000000000000000000 ) ) ;
#19990=AXIS2_PLACEMENT_3D ( 'NONE', #15215, #8011, #49438 ) ;
#20043=CARTESIAN_POINT ( 'NONE',  ( -23.50000000000000000, -13.25000000000000888, 32.75000000000000000 ) ) ;
#20115=VECTOR ( 'NONE', #33356, 1000.000000000000000 ) ;
#20132=DIRECTION ( 'NONE',  ( 0.000000000000000000, 2.413528314402514090E-16, -1.000000000000000000 ) ) ;
#20143=ORIENTED_EDGE ( 'NONE', *, *, #57350, .T. ) ;
#20199=DIRECTION ( 'NONE',  ( 0.000000000000000000, -4.336808689942017736E-16, 1.000000000000000000 ) ) ;
#20226=CARTESIAN_POINT ( 'NONE',  ( 19.00000000000000000, 8.999999999999996447, 23.75000000000000000 ) ) ;
#20285=CARTESIAN_POINT ( 'NONE',  ( 24.00000000000000000, 5.000000000000023093, 28.74999999999999645 ) ) ;
#20286=ORIENTED_EDGE ( 'NONE', *, *, #26687, .T. ) ;
#20374=CARTESIAN_POINT ( 'NONE',  ( 25.00000000000000711, -9.999999999999957367, 3.000000000000000000 ) ) ;
#20436=FACE_OUTER_BOUND ( 'NONE', #17417, .T. ) ;
#20450=CARTESIAN_POINT ( 'NONE',  ( -3.148799926473854982E-16, -1.749999999999995559, 32.75000000000000000 ) ) ;
#20499=EDGE_LOOP ( 'NONE', ( #32129, #9638, #52720, #46190, #72294, #21600 ) ) ;
#20789=AXIS2_PLACEMENT_3D ( 'NONE', #87333, #26502, #80572 ) ;
#20816=EDGE_CURVE ( 'NONE', #44546, #61438, #41787, .T. ) ;
#20835=ORIENTED_EDGE ( 'NONE', *, *, #80670, .T. ) ;
#20849=DIRECTION ( 'NONE',  ( -1.000000000000000000, 0.000000000000000000, 0.000000000000000000 ) ) ;
#20867=ORIENTED_EDGE ( 'NONE', *, *, #34345, .F. ) ;
#20879=ORIENTED_EDGE ( 'NONE', *, *, #13820, .T. ) ;
#20909=DIRECTION ( 'NONE',  ( -0.000000000000000000, -1.000000000000000000, 8.673617379884028076E-17 ) ) ;
#20912=ORIENTED_EDGE ( 'NONE', *, *, #41392, .T. ) ;
#20970=DIRECTION ( 'NONE',  ( 0.000000000000000000, -5.102127870520020612E-17, -1.000000000000000000 ) ) ;
#21017=DIRECTION ( 'NONE',  ( -0.000000000000000000, -5.102127870520021228E-17, -1.000000000000000000 ) ) ;
#21024=ORIENTED_EDGE ( 'NONE', *, *, #78582, .F. ) ;
#21087=EDGE_CURVE ( 'NONE', #6010, #15849, #25239, .T. ) ;
#21115=FACE_OUTER_BOUND ( 'NONE', #87965, .T. ) ;
#21176=CARTESIAN_POINT ( 'NONE',  ( -19.00000000000000000, -1.249999999999999334, 30.25000000000000000 ) ) ;
#21237=VECTOR ( 'NONE', #11610, 1000.000000000000000 ) ;
#21363=CARTESIAN_POINT ( 'NONE',  ( -19.00000000000000355, 12.75000000000004974, 30.81664701255125394 ) ) ;
#21405=DIRECTION ( 'NONE',  ( -0.000000000000000000, -0.000000000000000000, 1.000000000000000000 ) ) ;
#21406=ADVANCED_FACE ( 'NONE', ( #40649 ), #48274, .F. ) ;
#21437=EDGE_CURVE ( 'NONE', #66225, #79431, #63561, .T. ) ;
#21475=CARTESIAN_POINT ( 'NONE',  ( -27.00000000000000000, 9.000000000000001776, 2.999999999999995559 ) ) ;
#21514=AXIS2_PLACEMENT_3D ( 'NONE', #46039, #66310, #23538 ) ;
#21533=ORIENTED_EDGE ( 'NONE', *, *, #30408, .F. ) ;
#21553=CARTESIAN_POINT ( 'NONE',  ( -23.50000000000000000, 4.710477821889702467E-15, 29.24999999999999289 ) ) ;
#21590=ORIENTED_EDGE ( 'NONE', *, *, #31636, .F. ) ;
#21591=DIRECTION ( 'NONE',  ( -2.602085213965214586E-16, 1.000000000000000000, 0.000000000000000000 ) ) ;
#21600=ORIENTED_EDGE ( 'NONE', *, *, #63620, .T. ) ;
#21649=COLOUR_RGB ( '', 0.09019608, 0.27058824, 0.51372549) ;
#21691=ADVANCED_FACE ( 'NONE', ( #69695 ), #68811, .T. ) ;
#21739=FACE_OUTER_BOUND ( 'NONE', #46081, .T. ) ;
#21786=DIRECTION ( 'NONE',  ( 0.000000000000000000, -0.000000000000000000, -1.000000000000000000 ) ) ;
#21806=ORIENTED_EDGE ( 'NONE', *, *, #34547, .T. ) ;
#21830=ORIENTED_EDGE ( 'NONE', *, *, #59924, .T. ) ;
#21917=EDGE_CURVE ( 'NONE', #11165, #64684, #86338, .T. ) ;
#21923=VERTEX_POINT ( 'NONE', #73246 ) ;
#21952=EDGE_CURVE ( 'NONE', #57828, #87883, #45940, .T. ) ;
#22006=CARTESIAN_POINT ( 'NONE',  ( -23.50000000000000000, 9.000000000000024869, 29.25000000000000000 ) ) ;
#22029=EDGE_CURVE ( 'NONE', #79431, #33821, #35705, .T. ) ;
#22040=DIRECTION ( 'NONE',  ( -1.000000000000000000, -2.602085213965214586E-16, 0.000000000000000000 ) ) ;
#22043=CYLINDRICAL_SURFACE ( 'NONE', #85607, 8.000000000000000000 ) ;
#22131=EDGE_CURVE ( 'NONE', #63016, #67027, #31596, .T. ) ;
#22143=ORIENTED_EDGE ( 'NONE', *, *, #19098, .T. ) ;
#22203=CARTESIAN_POINT ( 'NONE',  ( -23.50000000000000000, 1.250000000000005329, 30.36437827766147279 ) ) ;
#22214=APPLICATION_CONTEXT ( 'automotive_design' ) ;
#22224=ADVANCED_FACE ( 'NONE', ( #23067 ), #53645, .T. ) ;
#22247=CARTESIAN_POINT ( 'NONE',  ( 25.00000000000000711, -9.999999999999957367, 13.00000000000000178 ) ) ;
#22280=PLANE ( 'NONE',  #24685 ) ;
#22349=LINE ( 'NONE', #15596, #64861 ) ;
#22477=DIRECTION ( 'NONE',  ( 0.000000000000000000, 0.000000000000000000, 1.000000000000000000 ) ) ;
#22538=ORIENTED_EDGE ( 'NONE', *, *, #71445, .T. ) ;
#22646=EDGE_CURVE ( 'NONE', #79547, #65630, #22914, .T. ) ;
#22724=EDGE_LOOP ( 'NONE', ( #37684, #23079, #19352, #16063 ) ) ;
#22732=CIRCLE ( 'NONE', #19912, 5.000000000000000888 ) ;
#22802=DIRECTION ( 'NONE',  ( -1.000000000000000000, -0.000000000000000000, -0.000000000000000000 ) ) ;
#22808=CARTESIAN_POINT ( 'NONE',  ( 25.00000000000000355, 9.999999999999971578, 13.00000000000000178 ) ) ;
#22850=DIRECTION ( 'NONE',  ( 0.000000000000000000, -1.000000000000000000, 0.000000000000000000 ) ) ;
#22887=EDGE_CURVE ( 'NONE', #33821, #78112, #14379, .T. ) ;
#22914=CIRCLE ( 'NONE', #86206, 6.614378277661484340 ) ;
#22915=CIRCLE ( 'NONE', #34436, 8.000000000000000000 ) ;
#23067=FACE_OUTER_BOUND ( 'NONE', #64989, .T. ) ;
#23079=ORIENTED_EDGE ( 'NONE', *, *, #27744, .F. ) ;
#23105=DIRECTION ( 'NONE',  ( -0.000000000000000000, -5.102127870520021228E-17, -1.000000000000000000 ) ) ;
#23113=CARTESIAN_POINT ( 'NONE',  ( -19.00000000000000000, -16.99999999999999645, 22.25000000000000355 ) ) ;
#23116=DIRECTION ( 'NONE',  ( 0.000000000000000000, 0.000000000000000000, -1.000000000000000000 ) ) ;
#23127=AXIS2_PLACEMENT_3D ( 'NONE', #31374, #24611, #59733 ) ;
#23144=ORIENTED_EDGE ( 'NONE', *, *, #21087, .F. ) ;
#23161=CARTESIAN_POINT ( 'NONE',  ( -24.00000000000000000, 9.000000000000024869, 29.25000000000000000 ) ) ;
#23354=VECTOR ( 'NONE', #23683, 1000.000000000000000 ) ;
#23359=ORIENTED_EDGE ( 'NONE', *, *, #34020, .T. ) ;
#23390=VERTEX_POINT ( 'NONE', #33949 ) ;
#23393=DIRECTION ( 'NONE',  ( -0.000000000000000000, -0.000000000000000000, 1.000000000000000000 ) ) ;
#23413=DIRECTION ( 'NONE',  ( 1.000000000000000000, -0.000000000000000000, -0.000000000000000000 ) ) ;
#23480=AXIS2_PLACEMENT_3D ( 'NONE', #54605, #19940, #87547 ) ;
#23538=DIRECTION ( 'NONE',  ( 0.000000000000000000, 1.084202172485504434E-16, -1.000000000000000000 ) ) ;
#23588=CARTESIAN_POINT ( 'NONE',  ( -23.50000000000000000, -9.499999999999982236, 27.74999999999999645 ) ) ;
#23609=CIRCLE ( 'NONE', #17841, 8.000000000000000000 ) ;
#23612=ORIENTED_EDGE ( 'NONE', *, *, #6428, .T. ) ;
#23676=CARTESIAN_POINT ( 'NONE',  ( 27.00000000000000000, -16.99999999999999645, 22.25000000000000355 ) ) ;
#23683=DIRECTION ( 'NONE',  ( 1.000000000000000000, -1.799314243699348838E-16, 0.000000000000000000 ) ) ;
#23773=EDGE_CURVE ( 'NONE', #67027, #15943, #67678, .T. ) ;
#23990=DIRECTION ( 'NONE',  ( 0.000000000000000000, 0.000000000000000000, 1.000000000000000000 ) ) ;
#24030=CARTESIAN_POINT ( 'NONE',  ( 19.99999999999996803, 15.00000000000000711, 13.00000000000000178 ) ) ;
#24133=FACE_OUTER_BOUND ( 'NONE', #25365, .T. ) ;
#24179=PLANE ( 'NONE',  #10198 ) ;
#24233=DIRECTION ( 'NONE',  ( -0.000000000000000000, -1.000000000000000000, 8.673617379884035472E-17 ) ) ;
#24274=EDGE_CURVE ( 'NONE', #56516, #76174, #66244, .T. ) ;
#24295=DIRECTION ( 'NONE',  ( -0.000000000000000000, 0.000000000000000000, -1.000000000000000000 ) ) ;
#24326=VERTEX_POINT ( 'NONE', #79499 ) ;
#24327=LINE ( 'NONE', #72525, #74342 ) ;
#24339=VECTOR ( 'NONE', #60884, 1000.000000000000000 ) ;
#24393=DIRECTION ( 'NONE',  ( -0.000000000000000000, -0.000000000000000000, -1.000000000000000000 ) ) ;
#24486=CARTESIAN_POINT ( 'NONE',  ( -25.00000000000000355, 9.999999999999971578, 13.00000000000000178 ) ) ;
#24496=DIRECTION ( 'NONE',  ( 0.000000000000000000, 0.000000000000000000, -1.000000000000000000 ) ) ;
#24611=DIRECTION ( 'NONE',  ( 1.000000000000000000, 1.734723475976812518E-16, -0.000000000000000000 ) ) ;
#24638=CARTESIAN_POINT ( 'NONE',  ( -24.00000000000000000, -5.499999999999981348, 27.75000000000000000 ) ) ;
#24663=LINE ( 'NONE', #18359, #28212 ) ;
#24685=AXIS2_PLACEMENT_3D ( 'NONE', #23161, #25385, #17294 ) ;
#24751=DIRECTION ( 'NONE',  ( 1.000000000000000000, 0.000000000000000000, -0.000000000000000000 ) ) ;
#24840=VECTOR ( 'NONE', #28347, 1000.000000000000000 ) ;
#24909=CARTESIAN_POINT ( 'NONE',  ( 27.00000000000000000, -1.249999999999999112, 32.75000000000000000 ) ) ;
#24955=ORIENTED_EDGE ( 'NONE', *, *, #2006, .F. ) ;
#24998=ORIENTED_EDGE ( 'NONE', *, *, #76662, .T. ) ;
#25016=LINE ( 'NONE', #45733, #86056 ) ;
#25020=DIRECTION ( 'NONE',  ( 1.000000000000000000, 0.000000000000000000, 0.000000000000000000 ) ) ;
#25030=STYLED_ITEM ( 'NONE', ( #71522 ), #29637 ) ;
#25046=ORIENTED_EDGE ( 'NONE', *, *, #74844, .F. ) ;
#25054=CARTESIAN_POINT ( 'NONE',  ( 27.00000000000000000, -8.999999999999996447, 22.25000000000000000 ) ) ;
#25105=CARTESIAN_POINT ( 'NONE',  ( -23.50000000000000000, 12.75000000000000355, 29.19862367942583603 ) ) ;
#25142=ORIENTED_EDGE ( 'NONE', *, *, #8750, .F. ) ;
#25224=VERTEX_POINT ( 'NONE', #33902 ) ;
#25239=CIRCLE ( 'NONE', #75566, 8.000000000000000000 ) ;
#25272=SPHERICAL_SURFACE ( 'NONE', #48040, 8.000000000000000000 ) ;
#25285=ORIENTED_EDGE ( 'NONE', *, *, #38205, .T. ) ;
#25324=EDGE_LOOP ( 'NONE', ( #47375, #6465, #52543, #36998 ) ) ;
#25365=EDGE_LOOP ( 'NONE', ( #41088, #41114, #80654, #40729 ) ) ;
#25380=ORIENTED_EDGE ( 'NONE', *, *, #369, .T. ) ;
#25381=ORIENTED_EDGE ( 'NONE', *, *, #85984, .T. ) ;
#25385=DIRECTION ( 'NONE',  ( 0.000000000000000000, 1.000000000000000000, -0.000000000000000000 ) ) ;
#25435=DIRECTION ( 'NONE',  ( 0.000000000000000000, 1.000000000000000000, 0.000000000000000000 ) ) ;
#25495=EDGE_CURVE ( 'NONE', #87883, #79547, #75006, .T. ) ;
#25496=DIRECTION ( 'NONE',  ( -0.000000000000000000, -1.000000000000000000, -0.000000000000000000 ) ) ;
#25499=DIRECTION ( 'NONE',  ( -0.000000000000000000, 5.102127870520020612E-17, 1.000000000000000000 ) ) ;
#25545=DIRECTION ( 'NONE',  ( 0.000000000000000000, -1.000000000000000000, -1.084202172485503448E-16 ) ) ;
#25546=ORIENTED_EDGE ( 'NONE', *, *, #1341, .T. ) ;
#25574=FACE_OUTER_BOUND ( 'NONE', #29296, .T. ) ;
#25629=( NAMED_UNIT ( * ) PLANE_ANGLE_UNIT ( ) SI_UNIT ( $, .RADIAN. ) );
#25686=CARTESIAN_POINT ( 'NONE',  ( -24.00000000000000000, 9.000000000000024869, 28.74999999999999645 ) ) ;
#25705=DIRECTION ( 'NONE',  ( 0.000000000000000000, 0.000000000000000000, -1.000000000000000000 ) ) ;
#25785=ADVANCED_FACE ( 'NONE', ( #58051 ), #37784, .T. ) ;
#25802=AXIS2_PLACEMENT_3D ( 'NONE', #26296, #53765, #26739 ) ;
#25859=ORIENTED_EDGE ( 'NONE', *, *, #11082, .T. ) ;
#25894=VECTOR ( 'NONE', #30569, 1000.000000000000000 ) ;
#25949=MECHANICAL_DESIGN_GEOMETRIC_PRESENTATION_REPRESENTATION('',(#79192),#40366);
#25952=DIRECTION ( 'NONE',  ( 1.000000000000000000, -0.000000000000000000, -0.000000000000000000 ) ) ;
#25970=CARTESIAN_POINT ( 'NONE',  ( -19.99999999999996447, -15.00000000000000533, 13.00000000000000178 ) ) ;
#26009=CIRCLE ( 'NONE', #37504, 8.000000000000000000 ) ;
#26020=DIRECTION ( 'NONE',  ( -1.000000000000000000, 0.000000000000000000, 0.000000000000000000 ) ) ;
#26121=ORIENTED_EDGE ( 'NONE', *, *, #22029, .F. ) ;
#26151=LINE ( 'NONE', #19393, #41647 ) ;
#26174=EDGE_CURVE ( 'NONE', #44526, #68629, #17416, .T. ) ;
#26176=CARTESIAN_POINT ( 'NONE',  ( -19.00000000000000000, -16.99999999999999289, 22.25000000000000000 ) ) ;
#26187=PLANE ( 'NONE',  #51913 ) ;
#26197=EDGE_LOOP ( 'NONE', ( #63824, #49549, #72030, #26483 ) ) ;
#26248=DIRECTION ( 'NONE',  ( 0.000000000000000000, -1.000000000000000000, -8.673617379884033500E-16 ) ) ;
#26268=VECTOR ( 'NONE', #45277, 1000.000000000000000 ) ;
#26290=DIRECTION ( 'NONE',  ( -1.734723475976813750E-16, 1.000000000000000000, -0.000000000000000000 ) ) ;
#26296=CARTESIAN_POINT ( 'NONE',  ( 27.00000000000000000, 0.7500000000000052180, 31.75000000000000000 ) ) ;
#26297=VECTOR ( 'NONE', #15585, 1000.000000000000000 ) ;
#26395=EDGE_CURVE ( 'NONE', #54784, #31550, #44829, .T. ) ;
#26403=CARTESIAN_POINT ( 'NONE',  ( -23.50000000000000000, 8.999999999999996447, 23.75000000000000000 ) ) ;
#26407=CARTESIAN_POINT ( 'NONE',  ( -23.50000000000000000, -16.99999999999999289, 28.86437827766147279 ) ) ;
#26409=ADVANCED_FACE ( 'NONE', ( #76342 ), #84010, .F. ) ;
#26483=ORIENTED_EDGE ( 'NONE', *, *, #21952, .T. ) ;
#26502=DIRECTION ( 'NONE',  ( -0.000000000000000000, -4.336808689942017243E-16, -1.000000000000000000 ) ) ;
#26600=CARTESIAN_POINT ( 'NONE',  ( 27.00000000000000000, 8.999999999999996447, 23.75000000000000000 ) ) ;
#26658=CARTESIAN_POINT ( 'NONE',  ( 24.00000000000000000, 5.000000000000023093, 29.24999999999999645 ) ) ;
#26683=ORIENTED_EDGE ( 'NONE', *, *, #48219, .F. ) ;
#26687=EDGE_CURVE ( 'NONE', #54790, #18166, #53752, .T. ) ;
#26701=CYLINDRICAL_SURFACE ( 'NONE', #23480, 8.000000000000000000 ) ;
#26739=DIRECTION ( 'NONE',  ( 0.000000000000000000, 1.084202172485503448E-16, -1.000000000000000000 ) ) ;
#26800=LINE ( 'NONE', #20043, #49400 ) ;
#26806=VERTEX_POINT ( 'NONE', #78339 ) ;
#26829=ORIENTED_EDGE ( 'NONE', *, *, #15624, .T. ) ;
#26885=DIRECTION ( 'NONE',  ( 1.845450506358306311E-16, -1.000000000000000000, 5.102127870520020612E-17 ) ) ;
#26930=CARTESIAN_POINT ( 'NONE',  ( -39.05038313613820122, -2.249999999999999556, 27.25000000000000000 ) ) ;
#26936=ORIENTED_EDGE ( 'NONE', *, *, #80257, .T. ) ;
#27018=CARTESIAN_POINT ( 'NONE',  ( 19.00000000000000000, 16.99999999999999289, 31.75000000000000000 ) ) ;
#27092=DIRECTION ( 'NONE',  ( 1.000000000000000000, -0.000000000000000000, -0.000000000000000000 ) ) ;
#27138=EDGE_CURVE ( 'NONE', #55802, #79573, #28741, .T. ) ;
#27158=DIRECTION ( 'NONE',  ( 0.000000000000000000, -8.673617379884028076E-17, -1.000000000000000000 ) ) ;
#27180=VECTOR ( 'NONE', #5872, 1000.000000000000000 ) ;
#27297=ORIENTED_EDGE ( 'NONE', *, *, #41392, .F. ) ;
#27306=LINE ( 'NONE', #44230, #15105 ) ;
#27348=LINE ( 'NONE', #35427, #37867 ) ;
#27590=DIRECTION ( 'NONE',  ( 0.000000000000000000, 2.546383084002652634E-16, 1.000000000000000000 ) ) ;
#27612=VECTOR ( 'NONE', #22850, 1000.000000000000000 ) ;
#27624=AXIS2_PLACEMENT_3D ( 'NONE', #65079, #3387, #38068 ) ;
#27737=CARTESIAN_POINT ( 'NONE',  ( 19.00000000000000000, 9.000000000000001776, 2.999999999999999556 ) ) ;
#27744=EDGE_CURVE ( 'NONE', #79573, #56516, #60535, .T. ) ;
#27812=LINE ( 'NONE', #48970, #47493 ) ;
#27820=CARTESIAN_POINT ( 'NONE',  ( 24.00000000000000000, 9.000000000000024869, 28.74999999999999645 ) ) ;
#27923=ORIENTED_EDGE ( 'NONE', *, *, #369, .F. ) ;
#27957=ORIENTED_EDGE ( 'NONE', *, *, #4128, .T. ) ;
#27967=CARTESIAN_POINT ( 'NONE',  ( -1.105886215935217678E-14, 12.75000000000002487, 13.00000000000000178 ) ) ;
#27980=LINE ( 'NONE', #68963, #60572 ) ;
#28024=ORIENTED_EDGE ( 'NONE', *, *, #88503, .T. ) ;
#28155=ORIENTED_EDGE ( 'NONE', *, *, #32573, .F. ) ;
#28190=CARTESIAN_POINT ( 'NONE',  ( 23.49999999999998934, 1.674711738930281374E-15, 13.00000000000000178 ) ) ;
#28212=VECTOR ( 'NONE', #52127, 1000.000000000000000 ) ;
#28232=EDGE_CURVE ( 'NONE', #76954, #31022, #48092, .T. ) ;
#28347=DIRECTION ( 'NONE',  ( -0.000000000000000000, -0.000000000000000000, -1.000000000000000000 ) ) ;
#28394=AXIS2_PLACEMENT_3D ( 'NONE', #355, #34131, #7555 ) ;
#28397=ORIENTED_EDGE ( 'NONE', *, *, #4874, .F. ) ;
#28400=CARTESIAN_POINT ( 'NONE',  ( 19.00000000000000000, -1.249999999999999334, 30.25000000000000000 ) ) ;
#28438=ORIENTED_EDGE ( 'NONE', *, *, #68324, .T. ) ;
#28590=VECTOR ( 'NONE', #19125, 1000.000000000000000 ) ;
#28603=VERTEX_POINT ( 'NONE', #84015 ) ;
#28741=LINE ( 'NONE', #16102, #27612 ) ;
#28742=CARTESIAN_POINT ( 'NONE',  ( -19.00000000000000000, 1.250000000000004663, 23.75000000000000000 ) ) ;
#28916=EDGE_LOOP ( 'NONE', ( #48130, #23144, #76515, #29524, #51054 ) ) ;
#28927=VECTOR ( 'NONE', #24393, 1000.000000000000000 ) ;
#28989=ORIENTED_EDGE ( 'NONE', *, *, #85460, .T. ) ;
#29001=DIRECTION ( 'NONE',  ( 0.000000000000000000, 0.000000000000000000, -1.000000000000000000 ) ) ;
#29028=FACE_OUTER_BOUND ( 'NONE', #3752, .T. ) ;
#29045=CARTESIAN_POINT ( 'NONE',  ( 27.00000000000000000, 0.000000000000000000, 24.75000000000000000 ) ) ;
#29054=FACE_OUTER_BOUND ( 'NONE', #39940, .T. ) ;
#29097=DIRECTION ( 'NONE',  ( -0.000000000000000000, 1.000000000000000000, -0.000000000000000000 ) ) ;
#29149=EDGE_CURVE ( 'NONE', #2479, #3057, #34997, .T. ) ;
#29296=EDGE_LOOP ( 'NONE', ( #18154, #16450, #39448, #34230 ) ) ;
#29350=AXIS2_PLACEMENT_3D ( 'NONE', #11270, #38743, #66207 ) ;
#29400=CARTESIAN_POINT ( 'NONE',  ( 20.00000000000000355, 10.00000000000000533, 13.00000000000000178 ) ) ;
#29440=CARTESIAN_POINT ( 'NONE',  ( 19.00000000000000000, -16.99999999999999289, 30.25000000000000000 ) ) ;
#29444=CARTESIAN_POINT ( 'NONE',  ( -24.00000000000000000, 9.000000000000024869, 28.74999999999999645 ) ) ;
#29491=EDGE_CURVE ( 'NONE', #16480, #38892, #81965, .T. ) ;
#29499=CARTESIAN_POINT ( 'NONE',  ( 27.00000000000000000, -1.249999999999999112, 32.75000000000000000 ) ) ;
#29524=ORIENTED_EDGE ( 'NONE', *, *, #60367, .T. ) ;
#29556=CARTESIAN_POINT ( 'NONE',  ( 19.00000000000000000, 16.99999999999999645, 23.75000000000000355 ) ) ;
#29579=CARTESIAN_POINT ( 'NONE',  ( 24.00000000000000000, 9.000000000000024869, 29.25000000000000000 ) ) ;
#29637=MANIFOLD_SOLID_BREP ( 'Cavity2', #80432 ) ;
#29641=CARTESIAN_POINT ( 'NONE',  ( 24.00000000000000000, 9.000000000000024869, 29.25000000000000000 ) ) ;
#29666=SURFACE_SIDE_STYLE ('',( #78277 ) ) ;
#29729=CARTESIAN_POINT ( 'NONE',  ( -19.00000000000000000, -13.25000000000000533, 22.25000000000000000 ) ) ;
#29745=DIRECTION ( 'NONE',  ( 0.000000000000000000, 0.000000000000000000, -1.000000000000000000 ) ) ;
#29777=CARTESIAN_POINT ( 'NONE',  ( -19.00000000000000000, 0.7500000000000052180, 31.75000000000000000 ) ) ;
#29870=EDGE_CURVE ( 'NONE', #79573, #65630, #68191, .T. ) ;
#29900=DIRECTION ( 'NONE',  ( 1.799314243699348838E-16, 1.000000000000000000, -5.102127870520020612E-17 ) ) ;
#29909=CARTESIAN_POINT ( 'NONE',  ( -23.50000000000000000, 5.000000000000023093, 28.74999999999999645 ) ) ;
#29937=DIRECTION ( 'NONE',  ( 0.000000000000000000, -1.000000000000000000, 0.000000000000000000 ) ) ;
#29947=AXIS2_PLACEMENT_3D ( 'NONE', #42314, #69767, #1305 ) ;
#29993=CARTESIAN_POINT ( 'NONE',  ( -24.00000000000000000, -9.499999999999982236, 27.74999999999999645 ) ) ;
#30034=VECTOR ( 'NONE', #9446, 1000.000000000000000 ) ;
#30157=CARTESIAN_POINT ( 'NONE',  ( -19.99999999999996447, -15.00000000000000533, 13.00000000000000178 ) ) ;
#30164=FACE_OUTER_BOUND ( 'NONE', #7437, .T. ) ;
#30165=CARTESIAN_POINT ( 'NONE',  ( -19.00000000000000000, -17.00000000000000000, 2.999999999999997780 ) ) ;
#30197=EDGE_CURVE ( 'NONE', #14162, #1369, #36542, .T. ) ;
#30230=ORIENTED_EDGE ( 'NONE', *, *, #73537, .T. ) ;
#30238=VERTEX_POINT ( 'NONE', #64431 ) ;
#30250=ORIENTED_EDGE ( 'NONE', *, *, #15156, .F. ) ;
#30272=CARTESIAN_POINT ( 'NONE',  ( -27.00000000000000000, -1.250000000000001110, 22.25000000000000000 ) ) ;
#30288=DIRECTION ( 'NONE',  ( -1.000000000000000000, -0.000000000000000000, -0.000000000000000000 ) ) ;
#30393=CARTESIAN_POINT ( 'NONE',  ( 19.00000000000000000, -8.999999999999998224, 22.25000000000000000 ) ) ;
#30395=CARTESIAN_POINT ( 'NONE',  ( 23.49999999999998934, -5.499999999999981348, 27.75000000000000000 ) ) ;
#30408=EDGE_CURVE ( 'NONE', #54790, #34521, #65768, .T. ) ;
#30438=AXIS2_PLACEMENT_3D ( 'NONE', #69588, #34910, #13755 ) ;
#30446=CARTESIAN_POINT ( 'NONE',  ( 24.00000000000000000, -5.499999999999981348, 27.75000000000000000 ) ) ;
#30455=ORIENTED_EDGE ( 'NONE', *, *, #68324, .F. ) ;
#30468=VECTOR ( 'NONE', #31314, 1000.000000000000000 ) ;
#30536=ORIENTED_EDGE ( 'NONE', *, *, #34763, .F. ) ;
#30569=DIRECTION ( 'NONE',  ( -0.000000000000000000, -1.000000000000000000, -0.000000000000000000 ) ) ;
#30750=PLANE ( 'NONE',  #9076 ) ;
#30754=MECHANICAL_DESIGN_GEOMETRIC_PRESENTATION_REPRESENTATION('',(#25030),#32241);
#30776=EDGE_CURVE ( 'NONE', #65772, #56866, #38645, .T. ) ;
#30778=VECTOR ( 'NONE', #27158, 1000.000000000000000 ) ;
#31022=VERTEX_POINT ( 'NONE', #36756 ) ;
#31066=DIRECTION ( 'NONE',  ( -5.997714145664496128E-17, -1.000000000000000000, 5.102127870520020612E-17 ) ) ;
#31084=ORIENTED_EDGE ( 'NONE', *, *, #53045, .T. ) ;
#31127=DIRECTION ( 'NONE',  ( -1.845450506358306311E-16, 1.000000000000000000, -5.102127870520021228E-17 ) ) ;
#31139=EDGE_CURVE ( 'NONE', #45549, #57327, #62438, .T. ) ;
#31151=LINE ( 'NONE', #58623, #28927 ) ;
#31175=DIRECTION ( 'NONE',  ( 1.000000000000000000, -0.000000000000000000, -0.000000000000000000 ) ) ;
#31184=CARTESIAN_POINT ( 'NONE',  ( 0.000000000000000000, 1.535740489026526408E-15, 28.00000000000000000 ) ) ;
#31188=CARTESIAN_POINT ( 'NONE',  ( -19.00000000000000000, -1.250000000000000222, 24.75000000000000000 ) ) ;
#31201=CARTESIAN_POINT ( 'NONE',  ( 19.00000000000000000, -1.749999999999999334, 22.25000000000000000 ) ) ;
#31207=DIRECTION ( 'NONE',  ( 0.000000000000000000, -1.000000000000000000, 0.000000000000000000 ) ) ;
#31210=FACE_OUTER_BOUND ( 'NONE', #46680, .T. ) ;
#31225=EDGE_CURVE ( 'NONE', #23390, #4149, #26800, .T. ) ;
#31287=ADVANCED_FACE ( 'NONE', ( #61903 ), #218, .F. ) ;
#31314=DIRECTION ( 'NONE',  ( 0.000000000000000000, 1.000000000000000000, 8.673617379884034486E-16 ) ) ;
#31348=CIRCLE ( 'NONE', #81713, 5.000000000000000888 ) ;
#31374=CARTESIAN_POINT ( 'NONE',  ( -25.00000000000000355, 9.999999999999971578, 13.00000000000000178 ) ) ;
#31476=ORIENTED_EDGE ( 'NONE', *, *, #59237, .T. ) ;
#31481=VERTEX_POINT ( 'NONE', #45176 ) ;
#31490=CARTESIAN_POINT ( 'NONE',  ( 23.49999999999998934, 5.000000000000023093, 32.75000000000000000 ) ) ;
#31550=VERTEX_POINT ( 'NONE', #76542 ) ;
#31554=AXIS2_PLACEMENT_3D ( 'NONE', #26930, #54389, #69241 ) ;
#31578=EDGE_CURVE ( 'NONE', #15943, #38361, #54940, .T. ) ;
#31596=LINE ( 'NONE', #30272, #53139 ) ;
#31608=ADVANCED_FACE ( 'NONE', ( #83306 ), #83751, .T. ) ;
#31618=DIRECTION ( 'NONE',  ( 0.000000000000000000, 0.000000000000000000, 1.000000000000000000 ) ) ;
#31636=EDGE_CURVE ( 'NONE', #88176, #47159, #84639, .T. ) ;
#31702=ORIENTED_EDGE ( 'NONE', *, *, #57396, .F. ) ;
#31755=FACE_OUTER_BOUND ( 'NONE', #111, .T. ) ;
#31822=FACE_BOUND ( 'NONE', #66053, .T. ) ;
#32063=ORIENTED_EDGE ( 'NONE', *, *, #57350, .F. ) ;
#32120=LINE ( 'NONE', #2517, #23354 ) ;
#32129=ORIENTED_EDGE ( 'NONE', *, *, #31578, .T. ) ;
#32193=EDGE_CURVE ( 'NONE', #3057, #67027, #38099, .T. ) ;
#32225=ORIENTED_EDGE ( 'NONE', *, *, #39857, .T. ) ;
#32241=( GEOMETRIC_REPRESENTATION_CONTEXT ( 3 ) GLOBAL_UNCERTAINTY_ASSIGNED_CONTEXT ( ( #14577 ) ) GLOBAL_UNIT_ASSIGNED_CONTEXT ( ( #80064, #37741, #3504 ) ) REPRESENTATION_CONTEXT ( 'NONE', 'WORKASPACE' ) );
#32266=DIRECTION ( 'NONE',  ( 0.000000000000000000, -1.084202172485503448E-16, 1.000000000000000000 ) ) ;
#32279=DIRECTION ( 'NONE',  ( -0.000000000000000000, -1.000000000000000000, -0.000000000000000000 ) ) ;
#32308=ORIENTED_EDGE ( 'NONE', *, *, #53165, .T. ) ;
#32536=DIRECTION ( 'NONE',  ( -1.799314243699348838E-16, -1.000000000000000000, 5.102127870520021228E-17 ) ) ;
#32542=CARTESIAN_POINT ( 'NONE',  ( 23.49999999999998934, 1.674711738930281374E-15, 28.74999999999999645 ) ) ;
#32556=PLANE ( 'NONE',  #82509 ) ;
#32573=EDGE_CURVE ( 'NONE', #77030, #88830, #80332, .T. ) ;
#32605=PLANE ( 'NONE',  #25802 ) ;
#32709=LINE ( 'NONE', #26407, #7302 ) ;
#32711=VECTOR ( 'NONE', #78720, 1000.000000000000000 ) ;
#32740=LINE ( 'NONE', #60209, #85173 ) ;
#32742=CARTESIAN_POINT ( 'NONE',  ( 19.00000000000000000, 0.7500000000000061062, 23.75000000000000000 ) ) ;
#32757=ADVANCED_FACE ( 'NONE', ( #17591 ), #86503, .T. ) ;
#32798=VERTEX_POINT ( 'NONE', #79546 ) ;
#32839=LINE ( 'NONE', #47679, #44930 ) ;
#32892=ORIENTED_EDGE ( 'NONE', *, *, #47586, .T. ) ;
#32921=ORIENTED_EDGE ( 'NONE', *, *, #2006, .T. ) ;
#32923=ORIENTED_EDGE ( 'NONE', *, *, #11082, .F. ) ;
#32928=CARTESIAN_POINT ( 'NONE',  ( 23.49999999999998579, 8.999999999999996447, 30.36437827766148345 ) ) ;
#32949=FACE_OUTER_BOUND ( 'NONE', #76465, .T. ) ;
#33037=EDGE_CURVE ( 'NONE', #9922, #73822, #1557, .T. ) ;
#33093=ORIENTED_EDGE ( 'NONE', *, *, #58173, .T. ) ;
#33211=DIRECTION ( 'NONE',  ( 0.000000000000000000, 0.000000000000000000, -1.000000000000000000 ) ) ;
#33249=ADVANCED_FACE ( 'NONE', ( #40232 ), #39789, .F. ) ;
#33356=DIRECTION ( 'NONE',  ( -0.000000000000000000, 1.000000000000000000, -0.000000000000000000 ) ) ;
#33381=CARTESIAN_POINT ( 'NONE',  ( 19.00000000000000000, 0.000000000000000000, 23.75000000000000000 ) ) ;
#33391=ORIENTED_EDGE ( 'NONE', *, *, #11968, .F. ) ;
#33404=ORIENTED_EDGE ( 'NONE', *, *, #42491, .T. ) ;
#33495=CARTESIAN_POINT ( 'NONE',  ( -23.50000000000000000, 1.250000000000003775, 28.00000000000000000 ) ) ;
#33519=DIRECTION ( 'NONE',  ( 0.000000000000000000, -2.546383084002652634E-16, -1.000000000000000000 ) ) ;
#33609=DIRECTION ( 'NONE',  ( -1.000000000000000000, 0.000000000000000000, 0.000000000000000000 ) ) ;
#33636=ADVANCED_FACE ( 'NONE', ( #88334 ), #25272, .T. ) ;
#33720=( NAMED_UNIT ( * ) PLANE_ANGLE_UNIT ( ) SI_UNIT ( $, .RADIAN. ) );
#33727=CARTESIAN_POINT ( 'NONE',  ( 23.49999999999998934, 9.000000000000024869, 28.74999999999999645 ) ) ;
#33771=EDGE_CURVE ( 'NONE', #39, #7626, #41450, .T. ) ;
#33794=LINE ( 'NONE', #18953, #4339 ) ;
#33813=DIRECTION ( 'NONE',  ( 0.000000000000000000, 0.000000000000000000, -1.000000000000000000 ) ) ;
#33821=VERTEX_POINT ( 'NONE', #50401 ) ;
#33823=EDGE_CURVE ( 'NONE', #11728, #39, #55303, .T. ) ;
#33902=CARTESIAN_POINT ( 'NONE',  ( -17.76215049426127024, 12.75000000000001421, 13.00000000000000178 ) ) ;
#33949=CARTESIAN_POINT ( 'NONE',  ( -23.50000000000000000, -13.25000000000000533, 27.31828373317831549 ) ) ;
#33994=PLANE ( 'NONE',  #88238 ) ;
#34020=EDGE_CURVE ( 'NONE', #54784, #63016, #12180, .T. ) ;
#34131=DIRECTION ( 'NONE',  ( 8.673617379884044347E-16, -1.000000000000000000, 5.102127870520021228E-17 ) ) ;
#34156=SURFACE_STYLE_USAGE ( .BOTH. , #41364 ) ;
#34188=DIRECTION ( 'NONE',  ( 0.000000000000000000, 8.673617379884035472E-17, 1.000000000000000000 ) ) ;
#34229=FACE_OUTER_BOUND ( 'NONE', #12093, .T. ) ;
#34230=ORIENTED_EDGE ( 'NONE', *, *, #54286, .F. ) ;
#34240=CARTESIAN_POINT ( 'NONE',  ( -19.99999999999996447, -15.00000000000000533, 13.00000000000000178 ) ) ;
#34303=DIRECTION ( 'NONE',  ( 1.681660752236433198E-16, 1.000000000000000000, -5.102127870520021228E-17 ) ) ;
#34345=EDGE_CURVE ( 'NONE', #25224, #45114, #72604, .T. ) ;
#34406=CARTESIAN_POINT ( 'NONE',  ( -23.50000000000000000, -5.499999999999981348, 27.75000000000000000 ) ) ;
#34420=EDGE_LOOP ( 'NONE', ( #2700, #55701, #21806, #86991 ) ) ;
#34429=ADVANCED_FACE ( 'NONE', ( #21739 ), #77570, .T. ) ;
#34430=DIRECTION ( 'NONE',  ( 0.000000000000000000, -1.000000000000000000, 0.000000000000000000 ) ) ;
#34436=AXIS2_PLACEMENT_3D ( 'NONE', #1444, #7762, #56389 ) ;
#34439=LINE ( 'NONE', #62779, #6245 ) ;
#34490=AXIS2_PLACEMENT_3D ( 'NONE', #16758, #51402, #18109 ) ;
#34521=VERTEX_POINT ( 'NONE', #3233 ) ;
#34547=EDGE_CURVE ( 'NONE', #52607, #66583, #48213, .T. ) ;
#34563=CIRCLE ( 'NONE', #83507, 8.000000000000000000 ) ;
#34585=DIRECTION ( 'NONE',  ( 0.000000000000000000, -0.000000000000000000, -1.000000000000000000 ) ) ;
#34622=PLANE ( 'NONE',  #41016 ) ;
#34659=DIRECTION ( 'NONE',  ( -0.000000000000000000, 2.413528314402514090E-16, -1.000000000000000000 ) ) ;
#34763=EDGE_CURVE ( 'NONE', #23390, #31550, #56843, .T. ) ;
#34813=CARTESIAN_POINT ( 'NONE',  ( -18.23784950573857344, 12.75000000000000711, 30.81664701255125394 ) ) ;
#34866=DIRECTION ( 'NONE',  ( 0.000000000000000000, -0.000000000000000000, -1.000000000000000000 ) ) ;
#34868=ORIENTED_EDGE ( 'NONE', *, *, #18715, .T. ) ;
#34878=EDGE_CURVE ( 'NONE', #54784, #11728, #10782, .T. ) ;
#34910=DIRECTION ( 'NONE',  ( -1.000000000000000000, 0.000000000000000000, 0.000000000000000000 ) ) ;
#34970=VECTOR ( 'NONE', #1523, 1000.000000000000000 ) ;
#34997=CIRCLE ( 'NONE', #66648, 8.000000000000000000 ) ;
#35024=ORIENTED_EDGE ( 'NONE', *, *, #9454, .T. ) ;
#35098=AXIS2_PLACEMENT_3D ( 'NONE', #86557, #86101, #65371 ) ;
#35209=ORIENTED_EDGE ( 'NONE', *, *, #47419, .T. ) ;
#35270=ORIENTED_EDGE ( 'NONE', *, *, #47955, .T. ) ;
#35307=DIRECTION ( 'NONE',  ( 1.000000000000000000, 0.000000000000000000, 0.000000000000000000 ) ) ;
#35416=AXIS2_PLACEMENT_3D ( 'NONE', #81842, #75512, #20132 ) ;
#35427=CARTESIAN_POINT ( 'NONE',  ( -23.50000000000000000, -1.749999999999991118, 32.75000000000000000 ) ) ;
#35468=CARTESIAN_POINT ( 'NONE',  ( 24.00000000000000000, -5.499999999999981348, 27.75000000000000000 ) ) ;
#35509=DIRECTION ( 'NONE',  ( 0.000000000000000000, -4.336808689942017243E-16, 1.000000000000000000 ) ) ;
#35522=LINE ( 'NONE', #2165, #59671 ) ;
#35528=CARTESIAN_POINT ( 'NONE',  ( -25.00000000000000355, 9.999999999999971578, 13.00000000000000178 ) ) ;
#35540=ORIENTED_EDGE ( 'NONE', *, *, #5486, .F. ) ;
#35556=AXIS2_PLACEMENT_3D ( 'NONE', #69632, #8384, #82720 ) ;
#35597=DIRECTION ( 'NONE',  ( -0.000000000000000000, -5.102127870520021228E-17, -1.000000000000000000 ) ) ;
#35616=VERTEX_POINT ( 'NONE', #30395 ) ;
#35669=LINE ( 'NONE', #70334, #76041 ) ;
#35694=ORIENTED_EDGE ( 'NONE', *, *, #80430, .T. ) ;
#35697=DIRECTION ( 'NONE',  ( 1.000000000000000000, -1.799314243699348838E-16, 1.560656329602356967E-32 ) ) ;
#35705=LINE ( 'NONE', #56845, #35860 ) ;
#35842=DIRECTION ( 'NONE',  ( -1.000000000000000000, -0.000000000000000000, -0.000000000000000000 ) ) ;
#35860=VECTOR ( 'NONE', #1024, 1000.000000000000000 ) ;
#35868=PRODUCT_DEFINITION ( 'UNKNOWN', '', #11625, #50941 ) ;
#35885=ORIENTED_EDGE ( 'NONE', *, *, #26395, .T. ) ;
#35896=ADVANCED_FACE ( 'NONE', ( #12194 ), #87882, .F. ) ;
#35926=VECTOR ( 'NONE', #52986, 1000.000000000000000 ) ;
#35992=ADVANCED_FACE ( 'NONE', ( #34229 ), #71003, .F. ) ;
#36156=VECTOR ( 'NONE', #52228, 1000.000000000000000 ) ;
#36310=EDGE_LOOP ( 'NONE', ( #56055, #55239, #63625, #15312, #49628 ) ) ;
#36331=ORIENTED_EDGE ( 'NONE', *, *, #52559, .T. ) ;
#36427=VERTEX_POINT ( 'NONE', #70039 ) ;
#36435=CARTESIAN_POINT ( 'NONE',  ( 19.00000000000000000, -16.99999999999999645, 22.25000000000000355 ) ) ;
#36454=ORIENTED_EDGE ( 'NONE', *, *, #57396, .T. ) ;
#36482=DIRECTION ( 'NONE',  ( 1.000000000000000000, 0.000000000000000000, 0.000000000000000000 ) ) ;
#36535=CARTESIAN_POINT ( 'NONE',  ( -17.76215049426127024, 12.75000000000001599, 32.75000000000000000 ) ) ;
#36542=LINE ( 'NONE', #77520, #6341 ) ;
#36601=ORIENTED_EDGE ( 'NONE', *, *, #48347, .F. ) ;
#36602=DIRECTION ( 'NONE',  ( 0.000000000000000000, -1.000000000000000000, -4.336808689942017736E-16 ) ) ;
#36617=VECTOR ( 'NONE', #80193, 1000.000000000000000 ) ;
#36630=DIRECTION ( 'NONE',  ( -1.000000000000000000, 0.000000000000000000, -0.000000000000000000 ) ) ;
#36658=DIRECTION ( 'NONE',  ( 0.000000000000000000, 1.000000000000000000, 0.000000000000000000 ) ) ;
#36756=CARTESIAN_POINT ( 'NONE',  ( -19.99999999999996803, 15.00000000000000711, 3.000000000000000000 ) ) ;
#36842=CARTESIAN_POINT ( 'NONE',  ( 23.49999999999998579, 0.000000000000000000, 30.36437827766148345 ) ) ;
#36869=DIRECTION ( 'NONE',  ( -1.000000000000000000, -0.000000000000000000, -0.000000000000000000 ) ) ;
#36998=ORIENTED_EDGE ( 'NONE', *, *, #7321, .F. ) ;
#37071=CARTESIAN_POINT ( 'NONE',  ( -23.50000000000000000, 5.000000000000023093, 32.75000000000000000 ) ) ;
#37076=ORIENTED_EDGE ( 'NONE', *, *, #72866, .F. ) ;
#37307=AXIS2_PLACEMENT_3D ( 'NONE', #26176, #13110, #5019 ) ;
#37331=DIRECTION ( 'NONE',  ( 0.000000000000000000, -1.000000000000000000, 5.421010862427522170E-17 ) ) ;
#37492=LINE ( 'NONE', #45588, #3764 ) ;
#37504=AXIS2_PLACEMENT_3D ( 'NONE', #63710, #29937, #24496 ) ;
#37525=DIRECTION ( 'NONE',  ( 0.000000000000000000, 1.000000000000000000, -0.000000000000000000 ) ) ;
#37601=ORIENTED_EDGE ( 'NONE', *, *, #70774, .T. ) ;
#37617=FACE_OUTER_BOUND ( 'NONE', #22724, .T. ) ;
#37684=ORIENTED_EDGE ( 'NONE', *, *, #24274, .F. ) ;
#37741=( NAMED_UNIT ( * ) PLANE_ANGLE_UNIT ( ) SI_UNIT ( $, .RADIAN. ) );
#37751=DIRECTION ( 'NONE',  ( 1.000000000000000000, 2.602085213965214586E-16, 0.000000000000000000 ) ) ;
#37784=CYLINDRICAL_SURFACE ( 'NONE', #64890, 8.000000000000000000 ) ;
#37811=CARTESIAN_POINT ( 'NONE',  ( -27.00000000000000000, -8.999999999999996447, 22.25000000000000000 ) ) ;
#37863=DIRECTION ( 'NONE',  ( -0.000000000000000000, 0.000000000000000000, 1.000000000000000000 ) ) ;
#37867=VECTOR ( 'NONE', #21017, 1000.000000000000000 ) ;
#37885=LINE ( 'NONE', #64012, #51974 ) ;
#37911=EDGE_CURVE ( 'NONE', #46479, #11121, #82054, .T. ) ;
#37914=DIRECTION ( 'NONE',  ( -0.000000000000000000, 1.000000000000000000, -0.000000000000000000 ) ) ;
#37952=PLANE ( 'NONE',  #61509 ) ;
#37980=ORIENTED_EDGE ( 'NONE', *, *, #23773, .T. ) ;
#37981=CARTESIAN_POINT ( 'NONE',  ( -27.00000000000000000, 0.000000000000000000, 0.000000000000000000 ) ) ;
#38017=VECTOR ( 'NONE', #8767, 1000.000000000000000 ) ;
#38033=ORIENTED_EDGE ( 'NONE', *, *, #1341, .F. ) ;
#38068=DIRECTION ( 'NONE',  ( 0.000000000000000000, 1.000000000000000000, -2.546383084002652634E-16 ) ) ;
#38069=LINE ( 'NONE', #10602, #26297 ) ;
#38099=LINE ( 'NONE', #66909, #46577 ) ;
#38205=EDGE_CURVE ( 'NONE', #66225, #56583, #41849, .T. ) ;
#38237=ORIENTED_EDGE ( 'NONE', *, *, #2474, .F. ) ;
#38269=FACE_BOUND ( 'NONE', #25324, .T. ) ;
#38361=VERTEX_POINT ( 'NONE', #55129 ) ;
#38414=EDGE_LOOP ( 'NONE', ( #77162, #14394, #33404, #9108 ) ) ;
#38434=DIRECTION ( 'NONE',  ( -1.000000000000000000, -0.000000000000000000, -0.000000000000000000 ) ) ;
#38570=ADVANCED_BREP_SHAPE_REPRESENTATION ( '', ( #29637, #83448 ), #80635 ) ;
#38630=VECTOR ( 'NONE', #36869, 1000.000000000000000 ) ;
#38642=EDGE_CURVE ( 'NONE', #73914, #84701, #72184, .T. ) ;
#38645=LINE ( 'NONE', #87747, #55314 ) ;
#38658=ORIENTED_EDGE ( 'NONE', *, *, #9679, .F. ) ;
#38743=DIRECTION ( 'NONE',  ( 0.000000000000000000, 8.673617379884033500E-16, -1.000000000000000000 ) ) ;
#38884=EDGE_CURVE ( 'NONE', #21923, #25224, #8626, .T. ) ;
#38892=VERTEX_POINT ( 'NONE', #29777 ) ;
#38910=EDGE_CURVE ( 'NONE', #38361, #64945, #24327, .T. ) ;
#39027=FACE_OUTER_BOUND ( 'NONE', #56791, .T. ) ;
#39070=DIRECTION ( 'NONE',  ( 0.000000000000000000, 1.000000000000000000, -0.000000000000000000 ) ) ;
#39079=VECTOR ( 'NONE', #40255, 1000.000000000000000 ) ;
#39127=LINE ( 'NONE', #72891, #19191 ) ;
#39147=CARTESIAN_POINT ( 'NONE',  ( 24.00000000000000000, -5.499999999999981348, 27.75000000000000000 ) ) ;
#39192=ORIENTED_EDGE ( 'NONE', *, *, #39667, .T. ) ;
#39204=DIRECTION ( 'NONE',  ( 1.000000000000000000, -1.799314243699348838E-16, 0.000000000000000000 ) ) ;
#39293=CARTESIAN_POINT ( 'NONE',  ( 23.49999999999998934, 1.250000000000002220, 32.75000000000000000 ) ) ;
#39448=ORIENTED_EDGE ( 'NONE', *, *, #29149, .F. ) ;
#39658=CARTESIAN_POINT ( 'NONE',  ( 27.00000000000000000, -13.24999999999999822, 29.02772085586297734 ) ) ;
#39667=EDGE_CURVE ( 'NONE', #60483, #57327, #17081, .T. ) ;
#39668=ORIENTED_EDGE ( 'NONE', *, *, #60401, .F. ) ;
#39698=CARTESIAN_POINT ( 'NONE',  ( -19.00000000000000000, 8.999999999999996447, 23.75000000000000000 ) ) ;
#39701=CARTESIAN_POINT ( 'NONE',  ( -23.50000000000000000, -5.499999999999981348, 27.24999999999999645 ) ) ;
#39709=CARTESIAN_POINT ( 'NONE',  ( -24.00000000000000000, -5.499999999999981348, 27.25000000000000000 ) ) ;
#39724=ORIENTED_EDGE ( 'NONE', *, *, #31636, .T. ) ;
#39778=CARTESIAN_POINT ( 'NONE',  ( 20.00000000000000711, -9.999999999999994671, 13.00000000000000178 ) ) ;
#39789=PLANE ( 'NONE',  #19315 ) ;
#39857=EDGE_CURVE ( 'NONE', #18166, #30238, #15989, .T. ) ;
#39911=ORIENTED_EDGE ( 'NONE', *, *, #27744, .T. ) ;
#39940=EDGE_LOOP ( 'NONE', ( #87152, #8266, #5314, #10003 ) ) ;
#39964=CARTESIAN_POINT ( 'NONE',  ( 19.00000000000000000, -16.99999999999999289, 30.25000000000000000 ) ) ;
#40002=CARTESIAN_POINT ( 'NONE',  ( -25.00000000000000000, -10.00000000000000533, 13.00000000000000178 ) ) ;
#40098=ORIENTED_EDGE ( 'NONE', *, *, #12961, .T. ) ;
#40103=CARTESIAN_POINT ( 'NONE',  ( 20.00000000000000355, 10.00000000000000533, 3.000000000000000000 ) ) ;
#40165=DIRECTION ( 'NONE',  ( 1.000000000000000000, 0.000000000000000000, 0.000000000000000000 ) ) ;
#40210=ORIENTED_EDGE ( 'NONE', *, *, #58232, .F. ) ;
#40232=FACE_OUTER_BOUND ( 'NONE', #66826, .T. ) ;
#40255=DIRECTION ( 'NONE',  ( 0.000000000000000000, 0.000000000000000000, 1.000000000000000000 ) ) ;
#40261=DIRECTION ( 'NONE',  ( -1.000000000000000000, 0.000000000000000000, 0.000000000000000000 ) ) ;
#40279=CARTESIAN_POINT ( 'NONE',  ( -24.00000000000000000, 9.000000000000024869, 29.25000000000000000 ) ) ;
#40366=( GEOMETRIC_REPRESENTATION_CONTEXT ( 3 ) GLOBAL_UNCERTAINTY_ASSIGNED_CONTEXT ( ( #64461 ) ) GLOBAL_UNIT_ASSIGNED_CONTEXT ( ( #82359, #33720, #53986 ) ) REPRESENTATION_CONTEXT ( 'NONE', 'WORKASPACE' ) );
#40387=EDGE_LOOP ( 'NONE', ( #69143, #49513, #86435, #22538, #83871 ) ) ;
#40428=ORIENTED_EDGE ( 'NONE', *, *, #12529, .F. ) ;
#40463=VECTOR ( 'NONE', #11027, 1000.000000000000000 ) ;
#40649=FACE_OUTER_BOUND ( 'NONE', #84256, .T. ) ;
#40676=VECTOR ( 'NONE', #63897, 1000.000000000000000 ) ;
#40729=ORIENTED_EDGE ( 'NONE', *, *, #12961, .F. ) ;
#40770=VECTOR ( 'NONE', #57911, 1000.000000000000000 ) ;
#40800=ORIENTED_EDGE ( 'NONE', *, *, #12535, .T. ) ;
#40821=ORIENTED_EDGE ( 'NONE', *, *, #60369, .F. ) ;
#40842=DIRECTION ( 'NONE',  ( -0.000000000000000000, 1.000000000000000000, 0.000000000000000000 ) ) ;
#40865=ORIENTED_EDGE ( 'NONE', *, *, #18031, .F. ) ;
#40901=CARTESIAN_POINT ( 'NONE',  ( -23.50000000000000000, 9.000000000000024869, 32.75000000000000000 ) ) ;
#40909=ORIENTED_EDGE ( 'NONE', *, *, #58788, .F. ) ;
#40966=CARTESIAN_POINT ( 'NONE',  ( 23.49999999999999645, -1.749999999999996447, 28.00000000000000000 ) ) ;
#41015=VERTEX_POINT ( 'NONE', #24638 ) ;
#41016=AXIS2_PLACEMENT_3D ( 'NONE', #47240, #834, #69299 ) ;
#41023=ORIENTED_EDGE ( 'NONE', *, *, #9679, .T. ) ;
#41030=EDGE_CURVE ( 'NONE', #62505, #24326, #45794, .T. ) ;
#41088=ORIENTED_EDGE ( 'NONE', *, *, #55492, .F. ) ;
#41114=ORIENTED_EDGE ( 'NONE', *, *, #50596, .F. ) ;
#41140=CYLINDRICAL_SURFACE ( 'NONE', #66674, 5.000000000000000888 ) ;
#41165=DIRECTION ( 'NONE',  ( 1.799314243699348838E-16, 1.000000000000000000, -5.102127870520020612E-17 ) ) ;
#41180=CARTESIAN_POINT ( 'NONE',  ( 23.49999999999998579, 12.75000000000000711, 29.19862367942584314 ) ) ;
#41194=DIRECTION ( 'NONE',  ( 0.000000000000000000, -1.000000000000000000, 0.000000000000000000 ) ) ;
#41196=LINE ( 'NONE', #14608, #6996 ) ;
#41289=CARTESIAN_POINT ( 'NONE',  ( 24.00000000000000000, -9.499999999999982236, 27.74999999999999645 ) ) ;
#41309=VECTOR ( 'NONE', #58115, 1000.000000000000000 ) ;
#41332=ORIENTED_EDGE ( 'NONE', *, *, #63620, .F. ) ;
#41364=SURFACE_SIDE_STYLE ('',( #13883 ) ) ;
#41366=CARTESIAN_POINT ( 'NONE',  ( 24.00000000000000000, -5.499999999999981348, 27.75000000000000000 ) ) ;
#41392=EDGE_CURVE ( 'NONE', #65630, #14162, #58646, .T. ) ;
#41450=LINE ( 'NONE', #42347, #4981 ) ;
#41481=ORIENTED_EDGE ( 'NONE', *, *, #42491, .F. ) ;
#41574=AXIS2_PLACEMENT_3D ( 'NONE', #14613, #77196, #36658 ) ;
#41635=ADVANCED_FACE ( 'NONE', ( #64402 ), #50452, .F. ) ;
#41646=DIRECTION ( 'NONE',  ( -0.000000000000000000, -0.000000000000000000, -1.000000000000000000 ) ) ;
#41647=VECTOR ( 'NONE', #46419, 1000.000000000000000 ) ;
#41654=ORIENTED_EDGE ( 'NONE', *, *, #60401, .T. ) ;
#41720=LINE ( 'NONE', #28190, #51653 ) ;
#41787=LINE ( 'NONE', #74237, #78453 ) ;
#41804=CYLINDRICAL_SURFACE ( 'NONE', #19990, 8.000000000000000000 ) ;
#41811=CARTESIAN_POINT ( 'NONE',  ( 23.49999999999998579, -8.999999999999996447, 22.25000000000000000 ) ) ;
#41848=ORIENTED_EDGE ( 'NONE', *, *, #84638, .F. ) ;
#41849=LINE ( 'NONE', #35528, #84439 ) ;
#41878=AXIS2_PLACEMENT_3D ( 'NONE', #27737, #20970, #48442 ) ;
#41938=AXIS2_PLACEMENT_3D ( 'NONE', #50517, #84776, #8670 ) ;
#41972=ORIENTED_EDGE ( 'NONE', *, *, #65114, .F. ) ;
#42032=ORIENTED_EDGE ( 'NONE', *, *, #33823, .F. ) ;
#42074=AXIS2_PLACEMENT_3D ( 'NONE', #19360, #81076, #87852 ) ;
#42110=EDGE_CURVE ( 'NONE', #76174, #57828, #87269, .T. ) ;
#42260=DIRECTION ( 'NONE',  ( 1.000000000000000000, -5.421010862427522170E-17, 0.000000000000000000 ) ) ;
#42290=ORIENTED_EDGE ( 'NONE', *, *, #30776, .T. ) ;
#42314=CARTESIAN_POINT ( 'NONE',  ( 23.49999999999998579, 8.999999999999996447, 23.75000000000000000 ) ) ;
#42316=CARTESIAN_POINT ( 'NONE',  ( 27.00000000000000000, -9.000000000000001776, 2.999999999999999556 ) ) ;
#42347=CARTESIAN_POINT ( 'NONE',  ( -27.00000000000000000, 17.00000000000000000, 2.999999999999999112 ) ) ;
#42374=DIRECTION ( 'NONE',  ( -1.000000000000000000, -8.673617379884044347E-16, 0.000000000000000000 ) ) ;
#42434=AXIS2_PLACEMENT_3D ( 'NONE', #73737, #11580, #46687 ) ;
#42462=DIRECTION ( 'NONE',  ( 0.000000000000000000, 0.000000000000000000, 1.000000000000000000 ) ) ;
#42469=LINE ( 'NONE', #8240, #44695 ) ;
#42476=CARTESIAN_POINT ( 'NONE',  ( 19.00000000000000000, 1.250000000000002665, 31.75000000000000000 ) ) ;
#42491=EDGE_CURVE ( 'NONE', #26806, #32798, #45353, .T. ) ;
#42523=CARTESIAN_POINT ( 'NONE',  ( 19.00000000000000000, 16.99999999999999289, 31.75000000000000000 ) ) ;
#42529=ORIENTED_EDGE ( 'NONE', *, *, #72866, .T. ) ;
#42593=ORIENTED_EDGE ( 'NONE', *, *, #24274, .T. ) ;
#42870=LINE ( 'NONE', #8196, #44440 ) ;
#42946=AXIS2_PLACEMENT_3D ( 'NONE', #37981, #11394, #80311 ) ;
#42965=CARTESIAN_POINT ( 'NONE',  ( 27.00000000000000000, -1.250000000000000000, 22.25000000000000000 ) ) ;
#43004=VERTEX_POINT ( 'NONE', #34406 ) ;
#43010=DIRECTION ( 'NONE',  ( -1.000000000000000000, 1.897353801849632760E-16, -8.673617379884035472E-16 ) ) ;
#43171=ADVANCED_FACE ( 'NONE', ( #16351 ), #37952, .T. ) ;
#43198=CARTESIAN_POINT ( 'NONE',  ( 19.99999999999997158, -14.99999999999999467, 13.00000000000000178 ) ) ;
#43267=ORIENTED_EDGE ( 'NONE', *, *, #12775, .T. ) ;
#43299=ADVANCED_FACE ( 'NONE', ( #81950 ), #88718, .F. ) ;
#43300=DIRECTION ( 'NONE',  ( 0.000000000000000000, 1.000000000000000000, -8.673617379884028076E-17 ) ) ;
#43383=FACE_OUTER_BOUND ( 'NONE', #18582, .T. ) ;
#43494=EDGE_CURVE ( 'NONE', #28603, #15849, #45366, .T. ) ;
#43543=VECTOR ( 'NONE', #33519, 1000.000000000000000 ) ;
#43600=ORIENTED_EDGE ( 'NONE', *, *, #31225, .F. ) ;
#43667=VECTOR ( 'NONE', #10078, 1000.000000000000000 ) ;
#43711=VECTOR ( 'NONE', #50948, 1000.000000000000000 ) ;
#43739=DIRECTION ( 'NONE',  ( -0.000000000000000000, 1.000000000000000000, -0.000000000000000000 ) ) ;
#43785=CARTESIAN_POINT ( 'NONE',  ( -17.92071683142037486, 12.74206001580630954, 30.82086045927834661 ) ) ;
#43855=AXIS2_PLACEMENT_3D ( 'NONE', #49212, #76688, #42462 ) ;
#43877=VERTEX_POINT ( 'NONE', #78170 ) ;
#43961=CARTESIAN_POINT ( 'NONE',  ( 23.49999999999998579, -13.24999999999999822, 27.31828373317832970 ) ) ;
#44033=ORIENTED_EDGE ( 'NONE', *, *, #48219, .T. ) ;
#44043=SURFACE_STYLE_USAGE ( .BOTH. , #29666 ) ;
#44063=ORIENTED_EDGE ( 'NONE', *, *, #41030, .T. ) ;
#44093=CARTESIAN_POINT ( 'NONE',  ( -24.00000000000000000, -5.499999999999981348, 27.75000000000000000 ) ) ;
#44118=ORIENTED_EDGE ( 'NONE', *, *, #60369, .T. ) ;
#44187=ORIENTED_EDGE ( 'NONE', *, *, #26174, .T. ) ;
#44189=CARTESIAN_POINT ( 'NONE',  ( -3.148799926473854489E-16, -1.749999999999995781, 28.00000000000000000 ) ) ;
#44214=FACE_OUTER_BOUND ( 'NONE', #17131, .T. ) ;
#44230=CARTESIAN_POINT ( 'NONE',  ( -24.00000000000000000, -5.499999999999981348, 27.25000000000000000 ) ) ;
#44237=CARTESIAN_POINT ( 'NONE',  ( 24.00000000000000000, 5.000000000000023093, 29.24999999999999645 ) ) ;
#44255=DIRECTION ( 'NONE',  ( -1.000000000000000000, 1.897353801849632760E-16, -3.469446951953614189E-15 ) ) ;
#44267=ORIENTED_EDGE ( 'NONE', *, *, #18597, .T. ) ;
#44381=DIRECTION ( 'NONE',  ( 0.000000000000000000, 0.000000000000000000, 1.000000000000000000 ) ) ;
#44440=VECTOR ( 'NONE', #24233, 1000.000000000000000 ) ;
#44479=CARTESIAN_POINT ( 'NONE',  ( 24.00000000000000000, -9.499999999999982236, 27.74999999999999645 ) ) ;
#44526=VERTEX_POINT ( 'NONE', #80645 ) ;
#44546=VERTEX_POINT ( 'NONE', #4972 ) ;
#44653=ORIENTED_EDGE ( 'NONE', *, *, #8844, .T. ) ;
#44660=PLANE ( 'NONE',  #34490 ) ;
#44695=VECTOR ( 'NONE', #63164, 1000.000000000000000 ) ;
#44698=DIRECTION ( 'NONE',  ( -1.000000000000000000, 0.000000000000000000, 0.000000000000000000 ) ) ;
#44726=FACE_OUTER_BOUND ( 'NONE', #7740, .T. ) ;
#44757=AXIS2_PLACEMENT_3D ( 'NONE', #30393, #72262, #15999 ) ;
#44829=CIRCLE ( 'NONE', #30438, 8.000000000000000000 ) ;
#44878=CARTESIAN_POINT ( 'NONE',  ( 19.00000000000000000, 0.000000000000000000, 22.25000000000000000 ) ) ;
#44895=VECTOR ( 'NONE', #76425, 1000.000000000000000 ) ;
#44930=VECTOR ( 'NONE', #59860, 1000.000000000000000 ) ;
#44990=EDGE_CURVE ( 'NONE', #56583, #33821, #41196, .T. ) ;
#45051=DIRECTION ( 'NONE',  ( 1.000000000000000000, 0.000000000000000000, 0.000000000000000000 ) ) ;
#45071=ADVANCED_FACE ( 'NONE', ( #31210 ), #3740, .F. ) ;
#45114=VERTEX_POINT ( 'NONE', #59575 ) ;
#45121=ORIENTED_EDGE ( 'NONE', *, *, #68936, .T. ) ;
#45138=ORIENTED_EDGE ( 'NONE', *, *, #38642, .T. ) ;
#45171=DIRECTION ( 'NONE',  ( 1.000000000000000000, -0.000000000000000000, -0.000000000000000000 ) ) ;
#45176=CARTESIAN_POINT ( 'NONE',  ( 19.00000000000000000, 12.75000000000000711, 30.81664701255128236 ) ) ;
#45193=EDGE_LOOP ( 'NONE', ( #81251, #71374, #18755, #80935, #67503, #41972 ) ) ;
#45277=DIRECTION ( 'NONE',  ( -1.000000000000000000, 0.000000000000000000, 0.000000000000000000 ) ) ;
#45353=LINE ( 'NONE', #29641, #87845 ) ;
#45366=LINE ( 'NONE', #36842, #32711 ) ;
#45381=ORIENTED_EDGE ( 'NONE', *, *, #51021, .F. ) ;
#45438=ADVANCED_FACE ( 'NONE', ( #61715 ), #5905, .T. ) ;
#45449=SHAPE_REPRESENTATION ( 'Outer Protective Cap', ( #83448 ), #80635 ) ;
#45513=ORIENTED_EDGE ( 'NONE', *, *, #20816, .F. ) ;
#45549=VERTEX_POINT ( 'NONE', #913 ) ;
#45588=CARTESIAN_POINT ( 'NONE',  ( 25.00000000000000355, 9.999999999999971578, 3.000000000000000000 ) ) ;
#45601=VECTOR ( 'NONE', #15076, 1000.000000000000000 ) ;
#45616=EDGE_CURVE ( 'NONE', #62505, #78112, #84676, .T. ) ;
#45700=LINE ( 'NONE', #11479, #28590 ) ;
#45727=EDGE_LOOP ( 'NONE', ( #10943, #64229, #85187, #68648, #62124, #11777 ) ) ;
#45733=CARTESIAN_POINT ( 'NONE',  ( -23.50000000000000000, -5.499999999999981348, 32.75000000000000000 ) ) ;
#45736=CARTESIAN_POINT ( 'NONE',  ( 20.00000000000000711, -9.999999999999994671, 3.000000000000000000 ) ) ;
#45746=DIRECTION ( 'NONE',  ( -1.000000000000000000, -0.000000000000000000, -0.000000000000000000 ) ) ;
#45755=AXIS2_PLACEMENT_3D ( 'NONE', #19703, #73776, #88193 ) ;
#45770=DIRECTION ( 'NONE',  ( 1.000000000000000000, -1.799314243699348838E-16, 1.560656329602356967E-32 ) ) ;
#45794=LINE ( 'NONE', #25970, #35926 ) ;
#45823=ADVANCED_FACE ( 'NONE', ( #87342 ), #46334, .F. ) ;
#45830=ADVANCED_FACE ( 'NONE', ( #75569 ), #41804, .T. ) ;
#45845=VERTEX_POINT ( 'NONE', #14318 ) ;
#45871=CARTESIAN_POINT ( 'NONE',  ( -19.00000000000000000, -8.999999999999994671, 30.24999999999999645 ) ) ;
#45940=CIRCLE ( 'NONE', #68964, 8.000000000000000000 ) ;
#45970=CIRCLE ( 'NONE', #14284, 8.000000000000000000 ) ;
#46039=CARTESIAN_POINT ( 'NONE',  ( -19.00000000000000000, 0.7500000000000059952, 24.75000000000000000 ) ) ;
#46081=EDGE_LOOP ( 'NONE', ( #12737, #62543, #28397, #55598, #57569, #5367 ) ) ;
#46097=ORIENTED_EDGE ( 'NONE', *, *, #80430, .F. ) ;
#46190=ORIENTED_EDGE ( 'NONE', *, *, #58219, .T. ) ;
#46334=PLANE ( 'NONE',  #17086 ) ;
#46416=ORIENTED_EDGE ( 'NONE', *, *, #47419, .F. ) ;
#46419=DIRECTION ( 'NONE',  ( -0.000000000000000000, -1.000000000000000000, -8.673617379884033500E-16 ) ) ;
#46450=EDGE_LOOP ( 'NONE', ( #86597, #26683, #40821, #58762 ) ) ;
#46479=VERTEX_POINT ( 'NONE', #54202 ) ;
#46502=ORIENTED_EDGE ( 'NONE', *, *, #18680, .F. ) ;
#46577=VECTOR ( 'NONE', #3860, 1000.000000000000000 ) ;
#46680=EDGE_LOOP ( 'NONE', ( #44267, #44187, #9914, #60159, #36331 ) ) ;
#46684=EDGE_LOOP ( 'NONE', ( #46416, #54272, #24998, #31084 ) ) ;
#46687=DIRECTION ( 'NONE',  ( 0.000000000000000000, 0.000000000000000000, 1.000000000000000000 ) ) ;
#46708=VECTOR ( 'NONE', #22477, 1000.000000000000000 ) ;
#46782=ORIENTED_EDGE ( 'NONE', *, *, #58788, .T. ) ;
#46784=CARTESIAN_POINT ( 'NONE',  ( -20.00000000000000355, -10.00000000000000533, 13.00000000000000178 ) ) ;
#46826=ORIENTED_EDGE ( 'NONE', *, *, #21437, .F. ) ;
#46829=AXIS2_PLACEMENT_3D ( 'NONE', #61690, #48181, #16500 ) ;
#46997=EDGE_LOOP ( 'NONE', ( #11684, #63380, #55868, #86315 ) ) ;
#47026=DIRECTION ( 'NONE',  ( 0.000000000000000000, -1.000000000000000000, 5.421010862427522170E-17 ) ) ;
#47089=FACE_OUTER_BOUND ( 'NONE', #26197, .T. ) ;
#47159=VERTEX_POINT ( 'NONE', #23588 ) ;
#47240=CARTESIAN_POINT ( 'NONE',  ( -24.00000000000000000, 5.000000000000023093, 29.24999999999999645 ) ) ;
#47275=ORIENTED_EDGE ( 'NONE', *, *, #41030, .F. ) ;
#47366=CIRCLE ( 'NONE', #21514, 8.000000000000000000 ) ;
#47375=ORIENTED_EDGE ( 'NONE', *, *, #60564, .F. ) ;
#47381=EDGE_LOOP ( 'NONE', ( #20867, #48010, #57725, #25859 ) ) ;
#47419=EDGE_CURVE ( 'NONE', #177, #84975, #22732, .T. ) ;
#47445=DIRECTION ( 'NONE',  ( 0.000000000000000000, 0.000000000000000000, -1.000000000000000000 ) ) ;
#47491=VECTOR ( 'NONE', #66077, 1000.000000000000000 ) ;
#47493=VECTOR ( 'NONE', #7988, 1000.000000000000000 ) ;
#47495=CARTESIAN_POINT ( 'NONE',  ( -19.99999999999996803, 15.00000000000000711, 13.00000000000000178 ) ) ;
#47535=VECTOR ( 'NONE', #35697, 1000.000000000000000 ) ;
#47586=EDGE_CURVE ( 'NONE', #15849, #54731, #70252, .T. ) ;
#47620=CIRCLE ( 'NONE', #8793, 8.000000000000000000 ) ;
#47679=CARTESIAN_POINT ( 'NONE',  ( 24.00000000000000000, -5.499999999999981348, 27.25000000000000000 ) ) ;
#47680=DIRECTION ( 'NONE',  ( 0.000000000000000000, -1.000000000000000000, -0.000000000000000000 ) ) ;
#47749=DIRECTION ( 'NONE',  ( -1.000000000000000000, -0.000000000000000000, -0.000000000000000000 ) ) ;
#47751=ADVANCED_FACE ( 'NONE', ( #25574 ), #19266, .T. ) ;
#47821=DIRECTION ( 'NONE',  ( 1.000000000000000000, -2.454804199071658828E-16, -2.454804199071659026E-15 ) ) ;
#47872=ADVANCED_FACE ( 'NONE', ( #82742 ), #80760, .T. ) ;
#47900=CARTESIAN_POINT ( 'NONE',  ( -18.00000000000000000, 2.999999999999935163, 32.75000000000000000 ) ) ;
#47915=DIRECTION ( 'NONE',  ( 0.000000000000000000, -2.413528314402514090E-16, 1.000000000000000000 ) ) ;
#47955=EDGE_CURVE ( 'NONE', #81222, #3726, #67238, .T. ) ;
#48010=ORIENTED_EDGE ( 'NONE', *, *, #38884, .F. ) ;
#48017=CARTESIAN_POINT ( 'NONE',  ( 24.00000000000000000, 9.000000000000024869, 28.74999999999999645 ) ) ;
#48039=DIRECTION ( 'NONE',  ( 0.000000000000000000, -1.000000000000000000, 0.000000000000000000 ) ) ;
#48040=AXIS2_PLACEMENT_3D ( 'NONE', #66705, #53175, #68470 ) ;
#48082=DIRECTION ( 'NONE',  ( -0.000000000000000000, 1.000000000000000000, -0.000000000000000000 ) ) ;
#48092=LINE ( 'NONE', #83225, #52153 ) ;
#48105=FILL_AREA_STYLE ('',( #67511 ) ) ;
#48130=ORIENTED_EDGE ( 'NONE', *, *, #47586, .F. ) ;
#48181=DIRECTION ( 'NONE',  ( 0.000000000000000000, -8.673617379884033500E-16, 1.000000000000000000 ) ) ;
#48213=LINE ( 'NONE', #39709, #3614 ) ;
#48219=EDGE_CURVE ( 'NONE', #5646, #44546, #35669, .T. ) ;
#48274=PLANE ( 'NONE',  #15276 ) ;
#48317=EDGE_LOOP ( 'NONE', ( #40865, #75464, #52845, #5699 ) ) ;
#48347=EDGE_CURVE ( 'NONE', #88176, #66583, #81984, .T. ) ;
#48380=DIRECTION ( 'NONE',  ( 0.000000000000000000, 8.131516293641283255E-17, 1.000000000000000000 ) ) ;
#48442=DIRECTION ( 'NONE',  ( 0.000000000000000000, -1.000000000000000000, 5.421010862427522170E-17 ) ) ;
#48489=EDGE_CURVE ( 'NONE', #56373, #35616, #63892, .T. ) ;
#48552=AXIS2_PLACEMENT_3D ( 'NONE', #32742, #25545, #66074 ) ;
#48575=CARTESIAN_POINT ( 'NONE',  ( -18.23784950573857344, 12.75000000000000711, 32.75000000000000000 ) ) ;
#48749=CARTESIAN_POINT ( 'NONE',  ( -27.00000000000000000, 0.7500000000000051070, 24.75000000000000000 ) ) ;
#48819=DIRECTION ( 'NONE',  ( -0.000000000000000000, 1.000000000000000000, -0.000000000000000000 ) ) ;
#48856=CARTESIAN_POINT ( 'NONE',  ( -24.00000000000000000, 5.000000000000023093, 28.74999999999999645 ) ) ;
#48864=AXIS2_PLACEMENT_3D ( 'NONE', #67184, #31618, #40165 ) ;
#48903=ORIENTED_EDGE ( 'NONE', *, *, #32193, .T. ) ;
#48926=CARTESIAN_POINT ( 'NONE',  ( -23.50000000000000000, 5.000000000000023093, 29.24999999999999645 ) ) ;
#48937=ORIENTED_EDGE ( 'NONE', *, *, #70558, .F. ) ;
#48970=CARTESIAN_POINT ( 'NONE',  ( 2.144117459101453788E-15, 12.75000000000001066, 13.00000000000000178 ) ) ;
#49025=DIRECTION ( 'NONE',  ( 0.000000000000000000, 1.000000000000000000, 8.673617379884034486E-16 ) ) ;
#49035=DIRECTION ( 'NONE',  ( -0.000000000000000000, -0.000000000000000000, -1.000000000000000000 ) ) ;
#49101=LINE ( 'NONE', #15771, #64668 ) ;
#49186=ORIENTED_EDGE ( 'NONE', *, *, #50596, .T. ) ;
#49212=CARTESIAN_POINT ( 'NONE',  ( -19.00000000000000000, 16.99999999999999289, 23.75000000000000000 ) ) ;
#49219=VECTOR ( 'NONE', #37751, 1000.000000000000000 ) ;
#49268=ORIENTED_EDGE ( 'NONE', *, *, #64615, .F. ) ;
#49400=VECTOR ( 'NONE', #12400, 1000.000000000000000 ) ;
#49438=DIRECTION ( 'NONE',  ( 0.000000000000000000, 0.000000000000000000, -1.000000000000000000 ) ) ;
#49479=VECTOR ( 'NONE', #68363, 1000.000000000000000 ) ;
#49513=ORIENTED_EDGE ( 'NONE', *, *, #81274, .T. ) ;
#49518=FACE_OUTER_BOUND ( 'NONE', #88983, .T. ) ;
#49549=ORIENTED_EDGE ( 'NONE', *, *, #26395, .F. ) ;
#49552=PLANE ( 'NONE',  #87661 ) ;
#49567=AXIS2_PLACEMENT_3D ( 'NONE', #65409, #31175, #11815 ) ;
#49571=ORIENTED_EDGE ( 'NONE', *, *, #18954, .F. ) ;
#49626=ORIENTED_EDGE ( 'NONE', *, *, #66552, .T. ) ;
#49628=ORIENTED_EDGE ( 'NONE', *, *, #22646, .F. ) ;
#49654=ORIENTED_EDGE ( 'NONE', *, *, #29491, .F. ) ;
#49723=ADVANCED_FACE ( 'NONE', ( #14294 ), #61587, .T. ) ;
#49878=VECTOR ( 'NONE', #35842, 1000.000000000000000 ) ;
#50156=ORIENTED_EDGE ( 'NONE', *, *, #34345, .T. ) ;
#50262=CARTESIAN_POINT ( 'NONE',  ( 27.00000000000000000, -8.999999999999996447, 22.25000000000000000 ) ) ;
#50288=AXIS2_PLACEMENT_3D ( 'NONE', #5246, #17878, #33609 ) ;
#50306=CARTESIAN_POINT ( 'NONE',  ( 24.00000000000000000, -9.499999999999982236, 27.25000000000000000 ) ) ;
#50401=CARTESIAN_POINT ( 'NONE',  ( -25.00000000000000000, -10.00000000000000533, 3.000000000000000000 ) ) ;
#50452=PLANE ( 'NONE',  #77708 ) ;
#50493=EDGE_CURVE ( 'NONE', #3057, #64684, #55508, .T. ) ;
#50517=CARTESIAN_POINT ( 'NONE',  ( 19.00000000000000000, 0.7500000000000059952, 24.75000000000000000 ) ) ;
#50596=EDGE_CURVE ( 'NONE', #41015, #62484, #26151, .T. ) ;
#50608=VERTEX_POINT ( 'NONE', #73457 ) ;
#50609=PRODUCT_DEFINITION_SHAPE ( 'NONE', 'NONE',  #35868 ) ;
#50639=ORIENTED_EDGE ( 'NONE', *, *, #5316, .T. ) ;
#50660=EDGE_LOOP ( 'NONE', ( #70695, #50156, #81578, #9687, #46502, #51947 ) ) ;
#50693=ORIENTED_EDGE ( 'NONE', *, *, #22646, .T. ) ;
#50706=EDGE_CURVE ( 'NONE', #1675, #76030, #14864, .T. ) ;
#50941=PRODUCT_DEFINITION_CONTEXT ( 'detailed design', #22214, 'design' ) ;
#50948=DIRECTION ( 'NONE',  ( 0.000000000000000000, -1.000000000000000000, 0.000000000000000000 ) ) ;
#51021=EDGE_CURVE ( 'NONE', #58097, #25224, #27812, .T. ) ;
#51031=ORIENTED_EDGE ( 'NONE', *, *, #68936, .F. ) ;
#51054=ORIENTED_EDGE ( 'NONE', *, *, #1086, .T. ) ;
#51309=ORIENTED_EDGE ( 'NONE', *, *, #5316, .F. ) ;
#51338=CARTESIAN_POINT ( 'NONE',  ( -39.05038313613820122, -2.249999999999999556, 27.25000000000000000 ) ) ;
#51361=DIRECTION ( 'NONE',  ( 0.000000000000000000, 0.000000000000000000, 1.000000000000000000 ) ) ;
#51376=ORIENTED_EDGE ( 'NONE', *, *, #15156, .T. ) ;
#51402=DIRECTION ( 'NONE',  ( -1.000000000000000000, 0.000000000000000000, 0.000000000000000000 ) ) ;
#51453=LINE ( 'NONE', #39658, #81553 ) ;
#51472=EDGE_LOOP ( 'NONE', ( #45513, #26829, #49571, #8113, #6909, #20879, #76270, #59840 ) ) ;
#51571=CARTESIAN_POINT ( 'NONE',  ( 2.445221920924756368E-15, -13.25000000000000533, 13.00000000000000178 ) ) ;
#51631=CARTESIAN_POINT ( 'NONE',  ( -39.05038313613820122, 12.25000000000000711, 28.74999999999999645 ) ) ;
#51653=VECTOR ( 'NONE', #14242, 1000.000000000000000 ) ;
#51703=VECTOR ( 'NONE', #47749, 1000.000000000000000 ) ;
#51712=CARTESIAN_POINT ( 'NONE',  ( -23.50000000000000000, 16.99999999999999289, 30.36437827766147279 ) ) ;
#51719=CARTESIAN_POINT ( 'NONE',  ( 20.00000000000000711, -9.999999999999994671, 13.00000000000000178 ) ) ;
#51820=AXIS2_PLACEMENT_3D ( 'NONE', #25054, #18750, #74580 ) ;
#51901=AXIS2_PLACEMENT_3D ( 'NONE', #4272, #19564, #47026 ) ;
#51913=AXIS2_PLACEMENT_3D ( 'NONE', #41366, #68830, #7136 ) ;
#51917=ORIENTED_EDGE ( 'NONE', *, *, #3518, .F. ) ;
#51947=ORIENTED_EDGE ( 'NONE', *, *, #87746, .F. ) ;
#51974=VECTOR ( 'NONE', #51361, 1000.000000000000000 ) ;
#52010=VECTOR ( 'NONE', #21405, 1000.000000000000000 ) ;
#52013=LINE ( 'NONE', #64187, #30468 ) ;
#52032=EDGE_LOOP ( 'NONE', ( #71338, #14706, #45121, #14965 ) ) ;
#52043=ORIENTED_EDGE ( 'NONE', *, *, #42110, .T. ) ;
#52073=CARTESIAN_POINT ( 'NONE',  ( -27.00000000000000000, 0.7500000000000052180, 31.75000000000000000 ) ) ;
#52081=DIRECTION ( 'NONE',  ( -0.000000000000000000, -0.000000000000000000, -1.000000000000000000 ) ) ;
#52127=DIRECTION ( 'NONE',  ( 0.000000000000000000, 1.000000000000000000, -0.000000000000000000 ) ) ;
#52153=VECTOR ( 'NONE', #801, 1000.000000000000000 ) ;
#52192=ORIENTED_EDGE ( 'NONE', *, *, #75199, .F. ) ;
#52206=ADVANCED_FACE ( 'NONE', ( #3888 ), #10661, .T. ) ;
#52228=DIRECTION ( 'NONE',  ( 0.000000000000000000, -1.000000000000000000, 0.000000000000000000 ) ) ;
#52237=DIRECTION ( 'NONE',  ( -1.000000000000000000, 0.000000000000000000, 0.000000000000000000 ) ) ;
#52311=VERTEX_POINT ( 'NONE', #60610 ) ;
#52327=FACE_BOUND ( 'NONE', #72783, .T. ) ;
#52332=ORIENTED_EDGE ( 'NONE', *, *, #14033, .F. ) ;
#52363=DIRECTION ( 'NONE',  ( 0.000000000000000000, 0.000000000000000000, 1.000000000000000000 ) ) ;
#52495=DIRECTION ( 'NONE',  ( 0.000000000000000000, -8.673617379884033500E-16, 1.000000000000000000 ) ) ;
#52543=ORIENTED_EDGE ( 'NONE', *, *, #37911, .F. ) ;
#52559=EDGE_CURVE ( 'NONE', #38361, #4430, #59053, .T. ) ;
#52588=CARTESIAN_POINT ( 'NONE',  ( -23.50000000000000000, -1.749999999999991340, 28.86437827766147279 ) ) ;
#52607=VERTEX_POINT ( 'NONE', #11898 ) ;
#52672=ORIENTED_EDGE ( 'NONE', *, *, #76759, .T. ) ;
#52704=AXIS2_PLACEMENT_3D ( 'NONE', #31201, #32536, #44255 ) ;
#52720=ORIENTED_EDGE ( 'NONE', *, *, #64441, .F. ) ;
#52822=DIRECTION ( 'NONE',  ( 1.000000000000000000, 0.000000000000000000, -0.000000000000000000 ) ) ;
#52845=ORIENTED_EDGE ( 'NONE', *, *, #9454, .F. ) ;
#52850=EDGE_CURVE ( 'NONE', #65772, #21923, #56465, .T. ) ;
#52879=LINE ( 'NONE', #40279, #15976 ) ;
#52892=DIRECTION ( 'NONE',  ( 1.000000000000000000, 0.000000000000000000, 0.000000000000000000 ) ) ;
#52921=DIRECTION ( 'NONE',  ( 0.000000000000000000, 0.000000000000000000, -1.000000000000000000 ) ) ;
#52955=DIRECTION ( 'NONE',  ( 0.000000000000000000, -1.000000000000000000, 5.102127870520020612E-17 ) ) ;
#52986=DIRECTION ( 'NONE',  ( 1.000000000000000000, 2.602085213965214586E-16, 0.000000000000000000 ) ) ;
#53021=VECTOR ( 'NONE', #9442, 1000.000000000000000 ) ;
#53034=ORIENTED_EDGE ( 'NONE', *, *, #18597, .F. ) ;
#53045=EDGE_CURVE ( 'NONE', #5642, #84975, #31151, .T. ) ;
#53139=VECTOR ( 'NONE', #37914, 1000.000000000000000 ) ;
#53158=CARTESIAN_POINT ( 'NONE',  ( 23.49999999999998934, 9.000000000000024869, 32.75000000000000000 ) ) ;
#53165=EDGE_CURVE ( 'NONE', #72099, #7817, #47620, .T. ) ;
#53175=DIRECTION ( 'NONE',  ( -0.000000000000000000, 1.000000000000000000, 0.000000000000000000 ) ) ;
#53184=ADVANCED_FACE ( 'NONE', ( #1704 ), #26187, .T. ) ;
#53258=AXIS2_PLACEMENT_3D ( 'NONE', #51719, #78318, #59389 ) ;
#53314=ADVANCED_FACE ( 'NONE', ( #64717 ), #24179, .T. ) ;
#53324=DIRECTION ( 'NONE',  ( 1.000000000000000000, -0.000000000000000000, -0.000000000000000000 ) ) ;
#53383=AXIS2_PLACEMENT_3D ( 'NONE', #3359, #58753, #86248 ) ;
#53399=ORIENTED_EDGE ( 'NONE', *, *, #12070, .T. ) ;
#53401=VERTEX_POINT ( 'NONE', #79587 ) ;
#53418=CARTESIAN_POINT ( 'NONE',  ( -19.00000000000000000, 1.250000000000007327, 31.75000000000000000 ) ) ;
#53645=CYLINDRICAL_SURFACE ( 'NONE', #37307, 8.000000000000000000 ) ;
#53651=PRODUCT_CONTEXT ( 'NONE', #56140, 'mechanical' ) ;
#53675=ORIENTED_EDGE ( 'NONE', *, *, #58823, .T. ) ;
#53681=CARTESIAN_POINT ( 'NONE',  ( 27.00000000000000000, -1.249999999999999778, 24.75000000000000000 ) ) ;
#53752=LINE ( 'NONE', #6025, #39079 ) ;
#53765=DIRECTION ( 'NONE',  ( 0.000000000000000000, -1.000000000000000000, -1.084202172485503448E-16 ) ) ;
#53801=EDGE_CURVE ( 'NONE', #52607, #41015, #37885, .T. ) ;
#53931=CIRCLE ( 'NONE', #42434, 6.614378277661474570 ) ;
#53961=FACE_OUTER_BOUND ( 'NONE', #63357, .T. ) ;
#53986=( NAMED_UNIT ( * ) SI_UNIT ( $, .STERADIAN. ) SOLID_ANGLE_UNIT ( ) );
#54202=CARTESIAN_POINT ( 'NONE',  ( 23.49999999999998934, 5.000000000000023093, 29.24999999999999645 ) ) ;
#54247=PLANE ( 'NONE',  #12133 ) ;
#54256=DIRECTION ( 'NONE',  ( -1.681660752236433198E-16, -1.000000000000000000, 5.102127870520020612E-17 ) ) ;
#54260=ORIENTED_EDGE ( 'NONE', *, *, #21917, .F. ) ;
#54272=ORIENTED_EDGE ( 'NONE', *, *, #59237, .F. ) ;
#54286=EDGE_CURVE ( 'NONE', #61438, #2479, #32740, .T. ) ;
#54343=DIRECTION ( 'NONE',  ( 1.000000000000000000, 1.845450506358306311E-16, 0.000000000000000000 ) ) ;
#54389=DIRECTION ( 'NONE',  ( -0.000000000000000000, 0.000000000000000000, 1.000000000000000000 ) ) ;
#54455=CARTESIAN_POINT ( 'NONE',  ( 24.00000000000000000, -9.499999999999982236, 27.74999999999999645 ) ) ;
#54540=LINE ( 'NONE', #27967, #73157 ) ;
#54554=ADVANCED_FACE ( 'NONE', ( #37617 ), #16906, .T. ) ;
#54577=ORIENTED_EDGE ( 'NONE', *, *, #85984, .F. ) ;
#54588=VECTOR ( 'NONE', #35597, 1000.000000000000000 ) ;
#54605=CARTESIAN_POINT ( 'NONE',  ( -19.00000000000000000, 8.999999999999994671, 31.75000000000000000 ) ) ;
#54731=VERTEX_POINT ( 'NONE', #41180 ) ;
#54784=VERTEX_POINT ( 'NONE', #23113 ) ;
#54790=VERTEX_POINT ( 'NONE', #29444 ) ;
#54810=AXIS2_PLACEMENT_3D ( 'NONE', #4098, #31127, #65363 ) ;
#54863=DIRECTION ( 'NONE',  ( -1.000000000000000000, 0.000000000000000000, -0.000000000000000000 ) ) ;
#54870=ADVANCED_FACE ( 'NONE', ( #21115 ), #74754, .T. ) ;
#54884=FACE_OUTER_BOUND ( 'NONE', #12132, .T. ) ;
#54907=LINE ( 'NONE', #54455, #82872 ) ;
#54940=LINE ( 'NONE', #61682, #78133 ) ;
#54994=DIRECTION ( 'NONE',  ( 1.000000000000000000, 8.673617379884044347E-16, 0.000000000000000000 ) ) ;
#55062=CARTESIAN_POINT ( 'NONE',  ( 27.00000000000000000, -16.99999999999999289, 30.25000000000000000 ) ) ;
#55088=FACE_OUTER_BOUND ( 'NONE', #1213, .T. ) ;
#55123=CARTESIAN_POINT ( 'NONE',  ( -23.50000000000000000, -9.499999999999982236, 27.25000000000000000 ) ) ;
#55126=PLANE ( 'NONE',  #88071 ) ;
#55129=CARTESIAN_POINT ( 'NONE',  ( -19.00000000000000000, -1.749999999999990674, 30.25000000000000000 ) ) ;
#55144=ORIENTED_EDGE ( 'NONE', *, *, #64441, .T. ) ;
#55176=ORIENTED_EDGE ( 'NONE', *, *, #68396, .T. ) ;
#55239=ORIENTED_EDGE ( 'NONE', *, *, #21952, .F. ) ;
#55303=CIRCLE ( 'NONE', #16479, 8.000000000000000000 ) ;
#55314=VECTOR ( 'NONE', #26020, 1000.000000000000000 ) ;
#55339=CARTESIAN_POINT ( 'NONE',  ( 23.49999999999998934, 9.000000000000024869, 29.25000000000000000 ) ) ;
#55340=DIRECTION ( 'NONE',  ( -1.000000000000000000, -0.000000000000000000, -0.000000000000000000 ) ) ;
#55364=DIRECTION ( 'NONE',  ( -1.000000000000000000, 0.000000000000000000, 0.000000000000000000 ) ) ;
#55388=EDGE_LOOP ( 'NONE', ( #28155, #52332, #40210, #66211 ) ) ;
#55472=DIRECTION ( 'NONE',  ( 0.000000000000000000, 0.000000000000000000, -1.000000000000000000 ) ) ;
#55492=EDGE_CURVE ( 'NONE', #62484, #47159, #64644, .T. ) ;
#55508=LINE ( 'NONE', #48749, #20115 ) ;
#55598=ORIENTED_EDGE ( 'NONE', *, *, #13820, .F. ) ;
#55686=ORIENTED_EDGE ( 'NONE', *, *, #6461, .F. ) ;
#55701=ORIENTED_EDGE ( 'NONE', *, *, #53801, .F. ) ;
#55728=LINE ( 'NONE', #27820, #75880 ) ;
#55740=FACE_OUTER_BOUND ( 'NONE', #28916, .T. ) ;
#55751=SHAPE_REPRESENTATION_RELATIONSHIP ( 'NONE' , 'NONE' ,  #45449, #38570 ) ;
#55802=VERTEX_POINT ( 'NONE', #42965 ) ;
#55868=ORIENTED_EDGE ( 'NONE', *, *, #21437, .T. ) ;
#55914=DIRECTION ( 'NONE',  ( 0.000000000000000000, 8.131516293641283255E-17, 1.000000000000000000 ) ) ;
#55924=EDGE_CURVE ( 'NONE', #19020, #88839, #2836, .T. ) ;
#55960=CARTESIAN_POINT ( 'NONE',  ( -19.00000000000000000, -17.00000000000000000, 2.999999999999999112 ) ) ;
#56035=VECTOR ( 'NONE', #22802, 1000.000000000000000 ) ;
#56055=ORIENTED_EDGE ( 'NONE', *, *, #25495, .F. ) ;
#56069=EDGE_CURVE ( 'NONE', #30238, #80750, #82956, .T. ) ;
#56140=APPLICATION_CONTEXT ( 'automotive_design' ) ;
#56206=DIRECTION ( 'NONE',  ( 5.997714145664496128E-17, 1.000000000000000000, -5.102127870520021228E-17 ) ) ;
#56270=DIRECTION ( 'NONE',  ( 0.000000000000000000, -2.413528314402514090E-16, 1.000000000000000000 ) ) ;
#56274=ORIENTED_EDGE ( 'NONE', *, *, #33823, .T. ) ;
#56344=CARTESIAN_POINT ( 'NONE',  ( 25.00000000000000355, 9.999999999999971578, 3.000000000000000000 ) ) ;
#56373=VERTEX_POINT ( 'NONE', #5421 ) ;
#56389=DIRECTION ( 'NONE',  ( 1.000000000000000000, -5.421010862427522170E-17, 2.602085213965210642E-15 ) ) ;
#56430=VECTOR ( 'NONE', #52363, 1000.000000000000000 ) ;
#56446=ORIENTED_EDGE ( 'NONE', *, *, #43494, .F. ) ;
#56465=B_SPLINE_CURVE_WITH_KNOTS ( 'NONE', 3,
 ( #70831, #71247, #43785, #1480 ),
 .UNSPECIFIED., .F., .F.,
 ( 4, 4 ),
 ( 0.000000000000000000, 0.0004756990114773013145 ),
 .UNSPECIFIED. ) ;
#56516=VERTEX_POINT ( 'NONE', #42316 ) ;
#56567=PLANE ( 'NONE',  #62287 ) ;
#56578=CARTESIAN_POINT ( 'NONE',  ( -17.76215049426128445, -1.749999999999992450, 30.25000000000000000 ) ) ;
#56579=EDGE_CURVE ( 'NONE', #57828, #54784, #65992, .T. ) ;
#56583=VERTEX_POINT ( 'NONE', #72309 ) ;
#56739=CARTESIAN_POINT ( 'NONE',  ( 25.00000000000000711, -9.999999999999957367, 13.00000000000000178 ) ) ;
#56791=EDGE_LOOP ( 'NONE', ( #50639, #56274, #81372, #2532, #54577, #70434, #57928, #42593 ) ) ;
#56803=DIRECTION ( 'NONE',  ( 1.734723475976812518E-16, -1.000000000000000000, 0.000000000000000000 ) ) ;
#56843=CIRCLE ( 'NONE', #64035, 6.777720855862973792 ) ;
#56845=CARTESIAN_POINT ( 'NONE',  ( -25.00000000000000000, -10.00000000000000533, 13.00000000000000178 ) ) ;
#56866=VERTEX_POINT ( 'NONE', #21363 ) ;
#56895=ADVANCED_FACE ( 'NONE', ( #29028 ), #3297, .T. ) ;
#57038=AXIS2_PLACEMENT_3D ( 'NONE', #75731, #34303, #47821 ) ;
#57145=CARTESIAN_POINT ( 'NONE',  ( 24.00000000000000000, -5.499999999999981348, 27.75000000000000000 ) ) ;
#57236=VECTOR ( 'NONE', #8791, 1000.000000000000000 ) ;
#57257=ORIENTED_EDGE ( 'NONE', *, *, #58232, .T. ) ;
#57327=VERTEX_POINT ( 'NONE', #20374 ) ;
#57350=EDGE_CURVE ( 'NONE', #67687, #55802, #67870, .T. ) ;
#57396=EDGE_CURVE ( 'NONE', #65802, #7817, #8636, .T. ) ;
#57529=ORIENTED_EDGE ( 'NONE', *, *, #17057, .T. ) ;
#57569=ORIENTED_EDGE ( 'NONE', *, *, #66552, .F. ) ;
#57597=CARTESIAN_POINT ( 'NONE',  ( -18.23784950573860186, -1.749999999999998668, 28.00000000000000355 ) ) ;
#57680=ORIENTED_EDGE ( 'NONE', *, *, #5486, .T. ) ;
#57689=PLANE ( 'NONE',  #5934 ) ;
#57691=DIRECTION ( 'NONE',  ( -0.000000000000000000, -5.102127870520021228E-17, -1.000000000000000000 ) ) ;
#57725=ORIENTED_EDGE ( 'NONE', *, *, #52850, .F. ) ;
#57828=VERTEX_POINT ( 'NONE', #36435 ) ;
#57860=CARTESIAN_POINT ( 'NONE',  ( -23.50000000000000000, 12.75000000000000355, 13.00000000000000178 ) ) ;
#57911=DIRECTION ( 'NONE',  ( -1.000000000000000000, -1.845450506358306311E-16, 0.000000000000000000 ) ) ;
#57921=EDGE_CURVE ( 'NONE', #78112, #45549, #18380, .T. ) ;
#57928=ORIENTED_EDGE ( 'NONE', *, *, #16116, .F. ) ;
#58011=AXIS2_PLACEMENT_3D ( 'NONE', #66792, #21591, #22040 ) ;
#58051=FACE_OUTER_BOUND ( 'NONE', #15985, .T. ) ;
#58097=VERTEX_POINT ( 'NONE', #1198 ) ;
#58111=CARTESIAN_POINT ( 'NONE',  ( -27.00000000000000000, -1.249999999999999778, 24.75000000000000000 ) ) ;
#58115=DIRECTION ( 'NONE',  ( -0.000000000000000000, 2.546383084002652634E-16, 1.000000000000000000 ) ) ;
#58173=EDGE_CURVE ( 'NONE', #85470, #7626, #84085, .T. ) ;
#58219=EDGE_CURVE ( 'NONE', #3688, #6905, #32120, .T. ) ;
#58222=CARTESIAN_POINT ( 'NONE',  ( -24.00000000000000000, 0.000000000000000000, 0.000000000000000000 ) ) ;
#58232=EDGE_CURVE ( 'NONE', #56373, #53401, #67243, .T. ) ;
#58444=ORIENTED_EDGE ( 'NONE', *, *, #70558, .T. ) ;
#58459=CARTESIAN_POINT ( 'NONE',  ( -23.50000000000000000, -9.499999999999982236, 32.75000000000000000 ) ) ;
#58506=VERTEX_POINT ( 'NONE', #2302 ) ;
#58543=CARTESIAN_POINT ( 'NONE',  ( -20.00000000000000355, 10.00000000000000711, 13.00000000000000178 ) ) ;
#58623=CARTESIAN_POINT ( 'NONE',  ( 19.99999999999996803, 15.00000000000000711, 13.00000000000000178 ) ) ;
#58646=LINE ( 'NONE', #59093, #10068 ) ;
#58648=LINE ( 'NONE', #39293, #10732 ) ;
#58658=DIRECTION ( 'NONE',  ( 0.000000000000000000, 8.131516293641283255E-17, 1.000000000000000000 ) ) ;
#58753=DIRECTION ( 'NONE',  ( -1.000000000000000000, 0.000000000000000000, 0.000000000000000000 ) ) ;
#58762=ORIENTED_EDGE ( 'NONE', *, *, #33037, .F. ) ;
#58788=EDGE_CURVE ( 'NONE', #24326, #45549, #19828, .T. ) ;
#58823=EDGE_CURVE ( 'NONE', #80750, #54790, #84203, .T. ) ;
#58952=LINE ( 'NONE', #59407, #3952 ) ;
#58997=CYLINDRICAL_SURFACE ( 'NONE', #77134, 5.000000000000000888 ) ;
#59053=CIRCLE ( 'NONE', #82089, 8.000000000000000000 ) ;
#59057=CARTESIAN_POINT ( 'NONE',  ( -19.00000000000000000, 0.7500000000000041078, 31.75000000000000000 ) ) ;
#59093=CARTESIAN_POINT ( 'NONE',  ( 23.49999999999998579, 0.000000000000000000, 28.86437827766148345 ) ) ;
#59132=CARTESIAN_POINT ( 'NONE',  ( -19.00000000000000000, 8.999999999999996447, 23.75000000000000000 ) ) ;
#59237=EDGE_CURVE ( 'NONE', #78849, #177, #69235, .T. ) ;
#59280=DIRECTION ( 'NONE',  ( 1.000000000000000000, -9.483446719664426957E-15, 0.000000000000000000 ) ) ;
#59348=ORIENTED_EDGE ( 'NONE', *, *, #7321, .T. ) ;
#59389=DIRECTION ( 'NONE',  ( -1.000000000000000000, 0.000000000000000000, 0.000000000000000000 ) ) ;
#59407=CARTESIAN_POINT ( 'NONE',  ( -19.00000000000000000, 16.99999999999999289, 31.75000000000000000 ) ) ;
#59456=ORIENTED_EDGE ( 'NONE', *, *, #27138, .F. ) ;
#59501=ORIENTED_EDGE ( 'NONE', *, *, #14490, .F. ) ;
#59535=CARTESIAN_POINT ( 'NONE',  ( -23.50000000000000000, 1.674711738930281374E-15, 32.75000000000000000 ) ) ;
#59575=CARTESIAN_POINT ( 'NONE',  ( -18.23784950573857344, 12.75000000000000888, 13.00000000000000178 ) ) ;
#59598=CARTESIAN_POINT ( 'NONE',  ( 19.00000000000000000, -1.249999999999999112, 32.75000000000000000 ) ) ;
#59657=SPHERICAL_SURFACE ( 'NONE', #76091, 8.000000000000000000 ) ;
#59671=VECTOR ( 'NONE', #55340, 1000.000000000000000 ) ;
#59705=LINE ( 'NONE', #87202, #8267 ) ;
#59733=DIRECTION ( 'NONE',  ( -1.734723475976812518E-16, 1.000000000000000000, 0.000000000000000000 ) ) ;
#59791=ADVANCED_FACE ( 'NONE', ( #60041 ), #26701, .T. ) ;
#59840=ORIENTED_EDGE ( 'NONE', *, *, #88340, .T. ) ;
#59860=DIRECTION ( 'NONE',  ( -1.000000000000000000, -0.000000000000000000, -0.000000000000000000 ) ) ;
#59924=EDGE_CURVE ( 'NONE', #84701, #35616, #39127, .T. ) ;
#59983=VECTOR ( 'NONE', #49025, 1000.000000000000000 ) ;
#60041=FACE_OUTER_BOUND ( 'NONE', #48317, .T. ) ;
#60045=ORIENTED_EDGE ( 'NONE', *, *, #48347, .T. ) ;
#60159=ORIENTED_EDGE ( 'NONE', *, *, #38910, .F. ) ;
#60173=DIRECTION ( 'NONE',  ( 0.000000000000000000, 1.835858764360065031E-15, 1.000000000000000000 ) ) ;
#60209=CARTESIAN_POINT ( 'NONE',  ( -19.00000000000000000, -1.249999999999999334, 32.75000000000000000 ) ) ;
#60216=CARTESIAN_POINT ( 'NONE',  ( 2.445221920924756368E-15, -13.25000000000000355, 32.75000000000000000 ) ) ;
#60363=ORIENTED_EDGE ( 'NONE', *, *, #43494, .T. ) ;
#60367=EDGE_CURVE ( 'NONE', #3726, #31481, #23609, .T. ) ;
#60369=EDGE_CURVE ( 'NONE', #73822, #5646, #73909, .T. ) ;
#60401=EDGE_CURVE ( 'NONE', #6010, #45845, #14606, .T. ) ;
#60403=SHAPE_DEFINITION_REPRESENTATION ( #50609, #45449 ) ;
#60433=ADVANCED_FACE ( 'NONE', ( #88514 ), #54247, .T. ) ;
#60483=VERTEX_POINT ( 'NONE', #22247 ) ;
#60535=LINE ( 'NONE', #6048, #43543 ) ;
#60564=EDGE_CURVE ( 'NONE', #17125, #76030, #73092, .T. ) ;
#60572=VECTOR ( 'NONE', #27092, 1000.000000000000000 ) ;
#60577=CARTESIAN_POINT ( 'NONE',  ( -23.50000000000000000, 1.674711738930281374E-15, 28.74999999999999645 ) ) ;
#60610=CARTESIAN_POINT ( 'NONE',  ( 23.49999999999998579, -13.25000000000000178, 13.00000000000000178 ) ) ;
#60628=AXIS2_PLACEMENT_3D ( 'NONE', #76159, #7271, #13141 ) ;
#60771=CARTESIAN_POINT ( 'NONE',  ( -27.00000000000000000, 0.7500000000000061062, 23.75000000000000000 ) ) ;
#60784=DIRECTION ( 'NONE',  ( -1.000000000000000000, -0.000000000000000000, -0.000000000000000000 ) ) ;
#60832=ORIENTED_EDGE ( 'NONE', *, *, #54286, .T. ) ;
#60839=DIRECTION ( 'NONE',  ( 0.000000000000000000, -1.000000000000000000, 0.000000000000000000 ) ) ;
#60884=DIRECTION ( 'NONE',  ( 0.000000000000000000, 0.000000000000000000, -1.000000000000000000 ) ) ;
#60963=EDGE_CURVE ( 'NONE', #423, #34521, #76460, .T. ) ;
#61040=ORIENTED_EDGE ( 'NONE', *, *, #31225, .T. ) ;
#61053=CYLINDRICAL_SURFACE ( 'NONE', #51820, 8.000000000000000000 ) ;
#61106=FACE_OUTER_BOUND ( 'NONE', #77089, .T. ) ;
#61137=ORIENTED_EDGE ( 'NONE', *, *, #76662, .F. ) ;
#61283=VECTOR ( 'NONE', #56803, 1000.000000000000000 ) ;
#61296=DIRECTION ( 'NONE',  ( 0.000000000000000000, 0.000000000000000000, 1.000000000000000000 ) ) ;
#61438=VERTEX_POINT ( 'NONE', #69505 ) ;
#61457=CARTESIAN_POINT ( 'NONE',  ( 2.144117459101453788E-15, 12.75000000000001243, 32.75000000000000000 ) ) ;
#61509=AXIS2_PLACEMENT_3D ( 'NONE', #44237, #8720, #64514 ) ;
#61587=PLANE ( 'NONE',  #31554 ) ;
#61639=CARTESIAN_POINT ( 'NONE',  ( 27.00000000000000000, 9.000000000000001776, 3.000000000000000444 ) ) ;
#61668=ADVANCED_FACE ( 'NONE', ( #52327, #79822, #73053 ), #66292, .F. ) ;
#61682=CARTESIAN_POINT ( 'NONE',  ( -19.00000000000000000, -16.99999999999999289, 30.25000000000000000 ) ) ;
#61690=CARTESIAN_POINT ( 'NONE',  ( -24.00000000000000000, 9.000000000000024869, 29.25000000000000000 ) ) ;
#61715=FACE_OUTER_BOUND ( 'NONE', #3466, .T. ) ;
#61903=FACE_OUTER_BOUND ( 'NONE', #14621, .T. ) ;
#61979=LINE ( 'NONE', #7496, #62716 ) ;
#62001=DIRECTION ( 'NONE',  ( 1.000000000000000000, -0.000000000000000000, -0.000000000000000000 ) ) ;
#62124=ORIENTED_EDGE ( 'NONE', *, *, #47955, .F. ) ;
#62135=CARTESIAN_POINT ( 'NONE',  ( -23.50000000000000000, 1.674711738930281374E-15, 27.25000000000000000 ) ) ;
#62139=ORIENTED_EDGE ( 'NONE', *, *, #39857, .F. ) ;
#62287=AXIS2_PLACEMENT_3D ( 'NONE', #41289, #40842, #84056 ) ;
#62438=CIRCLE ( 'NONE', #617, 5.000000000000000888 ) ;
#62484=VERTEX_POINT ( 'NONE', #18519 ) ;
#62503=EDGE_LOOP ( 'NONE', ( #37076, #65274, #57680, #71983 ) ) ;
#62505=VERTEX_POINT ( 'NONE', #34240 ) ;
#62513=DIRECTION ( 'NONE',  ( 0.000000000000000000, 1.000000000000000000, -8.673617379884028076E-17 ) ) ;
#62543=ORIENTED_EDGE ( 'NONE', *, *, #81392, .F. ) ;
#62544=CARTESIAN_POINT ( 'NONE',  ( 23.49999999999998934, -5.499999999999981348, 27.25000000000000000 ) ) ;
#62566=ORIENTED_EDGE ( 'NONE', *, *, #50493, .T. ) ;
#62610=DIRECTION ( 'NONE',  ( 1.000000000000000000, 2.559449574374560688E-16, -2.559449574374560589E-15 ) ) ;
#62716=VECTOR ( 'NONE', #23105, 1000.000000000000000 ) ;
#62763=CARTESIAN_POINT ( 'NONE',  ( 0.000000000000000000, 0.000000000000000000, 0.000000000000000000 ) ) ;
#62779=CARTESIAN_POINT ( 'NONE',  ( 27.00000000000000000, 0.7500000000000052180, 31.75000000000000000 ) ) ;
#62812=DIRECTION ( 'NONE',  ( 0.000000000000000000, 1.000000000000000000, -8.673617379884028076E-17 ) ) ;
#62869=LINE ( 'NONE', #68764, #64428 ) ;
#62877=ADVANCED_FACE ( 'NONE', ( #32949 ), #8138, .F. ) ;
#62955=FACE_OUTER_BOUND ( 'NONE', #34420, .T. ) ;
#63016=VERTEX_POINT ( 'NONE', #37811 ) ;
#63065=ORIENTED_EDGE ( 'NONE', *, *, #29870, .F. ) ;
#63164=DIRECTION ( 'NONE',  ( -1.000000000000000000, -0.000000000000000000, -0.000000000000000000 ) ) ;
#63175=ADVANCED_FACE ( 'NONE', ( #54884 ), #13448, .F. ) ;
#63357=EDGE_LOOP ( 'NONE', ( #12832, #17788, #23612, #25380 ) ) ;
#63380=ORIENTED_EDGE ( 'NONE', *, *, #38205, .F. ) ;
#63433=ORIENTED_EDGE ( 'NONE', *, *, #75862, .T. ) ;
#63525=DIRECTION ( 'NONE',  ( 0.000000000000000000, -1.000000000000000000, 5.421010862427522170E-17 ) ) ;
#63561=LINE ( 'NONE', #84301, #61283 ) ;
#63603=CARTESIAN_POINT ( 'NONE',  ( 19.00000000000000000, -8.999999999999996447, 22.25000000000000000 ) ) ;
#63607=DIRECTION ( 'NONE',  ( 0.000000000000000000, 0.000000000000000000, 1.000000000000000000 ) ) ;
#63620=EDGE_CURVE ( 'NONE', #67687, #15943, #3372, .T. ) ;
#63625=ORIENTED_EDGE ( 'NONE', *, *, #85635, .T. ) ;
#63641=ORIENTED_EDGE ( 'NONE', *, *, #73537, .F. ) ;
#63710=CARTESIAN_POINT ( 'NONE',  ( -19.00000000000000000, -8.999999999999996447, 22.25000000000000000 ) ) ;
#63736=ORIENTED_EDGE ( 'NONE', *, *, #2573, .F. ) ;
#63783=ORIENTED_EDGE ( 'NONE', *, *, #78582, .T. ) ;
#63790=LINE ( 'NONE', #29579, #56035 ) ;
#63792=VECTOR ( 'NONE', #60784, 1000.000000000000000 ) ;
#63814=ORIENTED_EDGE ( 'NONE', *, *, #30197, .T. ) ;
#63824=ORIENTED_EDGE ( 'NONE', *, *, #4128, .F. ) ;
#63827=ADVANCED_FACE ( 'NONE', ( #68196 ), #6495, .F. ) ;
#63863=ORIENTED_EDGE ( 'NONE', *, *, #65114, .T. ) ;
#63884=ORIENTED_EDGE ( 'NONE', *, *, #84638, .T. ) ;
#63892=LINE ( 'NONE', #57145, #38630 ) ;
#63897=DIRECTION ( 'NONE',  ( 0.000000000000000000, 1.000000000000000000, 0.000000000000000000 ) ) ;
#63920=CARTESIAN_POINT ( 'NONE',  ( -19.00000000000000000, -9.000000000000001776, 2.999999999999999112 ) ) ;
#64012=CARTESIAN_POINT ( 'NONE',  ( -24.00000000000000000, -5.499999999999981348, 27.75000000000000000 ) ) ;
#64035=AXIS2_PLACEMENT_3D ( 'NONE', #29729, #483, #62610 ) ;
#64108=CARTESIAN_POINT ( 'NONE',  ( -3.148799926473854982E-16, -1.749999999999995559, 32.75000000000000000 ) ) ;
#64122=CARTESIAN_POINT ( 'NONE',  ( -24.00000000000000000, 5.000000000000023093, 29.24999999999999645 ) ) ;
#64166=EDGE_CURVE ( 'NONE', #88839, #423, #841, .T. ) ;
#64187=CARTESIAN_POINT ( 'NONE',  ( -23.50000000000000000, 6.011520428872295955E-15, 27.75000000000000355 ) ) ;
#64229=ORIENTED_EDGE ( 'NONE', *, *, #52850, .T. ) ;
#64402=FACE_OUTER_BOUND ( 'NONE', #68378, .T. ) ;
#64428=VECTOR ( 'NONE', #62001, 1000.000000000000000 ) ;
#64431=CARTESIAN_POINT ( 'NONE',  ( -24.00000000000000000, 5.000000000000023093, 29.24999999999999645 ) ) ;
#64441=EDGE_CURVE ( 'NONE', #3688, #64945, #1023, .T. ) ;
#64461=UNCERTAINTY_MEASURE_WITH_UNIT (LENGTH_MEASURE( 1.000000000000000082E-05 ), #82359, 'distance_accuracy_value', 'NONE');
#64514=DIRECTION ( 'NONE',  ( 0.000000000000000000, -0.000000000000000000, 1.000000000000000000 ) ) ;
#64525=FACE_OUTER_BOUND ( 'NONE', #80770, .T. ) ;
#64539=ADVANCED_FACE ( 'NONE', ( #70078 ), #56567, .T. ) ;
#64572=AXIS2_PLACEMENT_3D ( 'NONE', #5821, #24751, #24295 ) ;
#64615=EDGE_CURVE ( 'NONE', #54731, #58097, #38069, .T. ) ;
#64644=LINE ( 'NONE', #29993, #75147 ) ;
#64658=LINE ( 'NONE', #51571, #40770 ) ;
#64668=VECTOR ( 'NONE', #23393, 1000.000000000000000 ) ;
#64684=VERTEX_POINT ( 'NONE', #8833 ) ;
#64717=FACE_OUTER_BOUND ( 'NONE', #81327, .T. ) ;
#64861=VECTOR ( 'NONE', #4179, 1000.000000000000000 ) ;
#64884=CIRCLE ( 'NONE', #44757, 8.000000000000000000 ) ;
#64890=AXIS2_PLACEMENT_3D ( 'NONE', #45871, #73354, #11661 ) ;
#64945=VERTEX_POINT ( 'NONE', #68210 ) ;
#64957=AXIS2_PLACEMENT_3D ( 'NONE', #29499, #62812, #82678 ) ;
#64961=DIRECTION ( 'NONE',  ( -1.734723475976813750E-16, 1.000000000000000000, -0.000000000000000000 ) ) ;
#64989=EDGE_LOOP ( 'NONE', ( #13869, #17925, #85389, #18036, #41848, #70037 ) ) ;
#64991=DIRECTION ( 'NONE',  ( 0.000000000000000000, 0.000000000000000000, 1.000000000000000000 ) ) ;
#65060=ADVANCED_FACE ( 'NONE', ( #64525 ), #30750, .F. ) ;
#65079=CARTESIAN_POINT ( 'NONE',  ( 19.00000000000000000, -9.000000000000001776, 2.291744775602387568E-15 ) ) ;
#65114=EDGE_CURVE ( 'NONE', #8219, #16365, #78493, .T. ) ;
#65182=DIRECTION ( 'NONE',  ( 0.000000000000000000, 0.000000000000000000, 1.000000000000000000 ) ) ;
#65247=CYLINDRICAL_SURFACE ( 'NONE', #53258, 5.000000000000000888 ) ;
#65274=ORIENTED_EDGE ( 'NONE', *, *, #56069, .F. ) ;
#65363=DIRECTION ( 'NONE',  ( 1.000000000000000000, 2.559449574374558716E-16, -5.118899148749117234E-15 ) ) ;
#65371=DIRECTION ( 'NONE',  ( -5.471219261342662483E-14, -1.000000000000000000, 0.000000000000000000 ) ) ;
#65409=CARTESIAN_POINT ( 'NONE',  ( -19.00000000000000000, 8.999999999999996447, 23.75000000000000000 ) ) ;
#65452=LINE ( 'NONE', #24909, #75297 ) ;
#65630=VERTEX_POINT ( 'NONE', #15654 ) ;
#65660=ADVANCED_FACE ( 'NONE', ( #82133 ), #41140, .F. ) ;
#65704=LINE ( 'NONE', #31490, #30034 ) ;
#65716=EDGE_CURVE ( 'NONE', #60483, #78849, #86794, .T. ) ;
#65718=VECTOR ( 'NONE', #47445, 1000.000000000000000 ) ;
#65749=ADVANCED_FACE ( 'NONE', ( #55088 ), #82584, .T. ) ;
#65768=LINE ( 'NONE', #25686, #36617 ) ;
#65772=VERTEX_POINT ( 'NONE', #34813 ) ;
#65802=VERTEX_POINT ( 'NONE', #42476 ) ;
#65880=DIRECTION ( 'NONE',  ( -1.000000000000000000, 1.799314243699348838E-16, 0.000000000000000000 ) ) ;
#65882=CARTESIAN_POINT ( 'NONE',  ( 27.00000000000000000, 16.99999999999999645, 23.75000000000000355 ) ) ;
#65899=AXIS2_PLACEMENT_3D ( 'NONE', #11544, #25499, #52955 ) ;
#65992=LINE ( 'NONE', #23676, #26268 ) ;
#66053=EDGE_LOOP ( 'NONE', ( #73568, #17740, #35209, #69391, #40800, #67029, #79493, #12528 ) ) ;
#66074=DIRECTION ( 'NONE',  ( 0.000000000000000000, 1.084202172485504434E-16, -1.000000000000000000 ) ) ;
#66077=DIRECTION ( 'NONE',  ( -0.000000000000000000, 2.546383084002652634E-16, 1.000000000000000000 ) ) ;
#66159=DIRECTION ( 'NONE',  ( 0.000000000000000000, -2.546383084002652634E-16, -1.000000000000000000 ) ) ;
#66173=PLANE ( 'NONE',  #64572 ) ;
#66207=DIRECTION ( 'NONE',  ( 0.000000000000000000, 1.000000000000000000, 8.673617379884033500E-16 ) ) ;
#66211=ORIENTED_EDGE ( 'NONE', *, *, #16138, .F. ) ;
#66225=VERTEX_POINT ( 'NONE', #24486 ) ;
#66244=CIRCLE ( 'NONE', #51901, 8.000000000000000000 ) ;
#66292=PLANE ( 'NONE',  #82658 ) ;
#66310=DIRECTION ( 'NONE',  ( -0.000000000000000000, 1.000000000000000000, 1.084202172485503448E-16 ) ) ;
#66336=EDGE_CURVE ( 'NONE', #73822, #55802, #67708, .T. ) ;
#66467=DIRECTION ( 'NONE',  ( 0.000000000000000000, -1.000000000000000000, -8.673617379884033500E-16 ) ) ;
#66486=EDGE_CURVE ( 'NONE', #67767, #68629, #66734, .T. ) ;
#66552=EDGE_CURVE ( 'NONE', #7817, #38892, #85213, .T. ) ;
#66583=VERTEX_POINT ( 'NONE', #39701 ) ;
#66617=DIRECTION ( 'NONE',  ( 0.000000000000000000, 0.000000000000000000, 1.000000000000000000 ) ) ;
#66648=AXIS2_PLACEMENT_3D ( 'NONE', #31188, #87499, #58658 ) ;
#66670=CARTESIAN_POINT ( 'NONE',  ( -23.50000000000000000, -13.25000000000001066, 13.00000000000000888 ) ) ;
#66674=AXIS2_PLACEMENT_3D ( 'NONE', #68167, #52081, #40261 ) ;
#66705=CARTESIAN_POINT ( 'NONE',  ( 19.00000000000000000, -8.999999999999996447, 22.25000000000000000 ) ) ;
#66734=CIRCLE ( 'NONE', #35098, 4.755951259987790891 ) ;
#66767=AXIS2_PLACEMENT_3D ( 'NONE', #5735, #48039, #33211 ) ;
#66792=CARTESIAN_POINT ( 'NONE',  ( -19.99999999999996447, -15.00000000000000533, 13.00000000000000178 ) ) ;
#66826=EDGE_LOOP ( 'NONE', ( #14969, #3658, #51309, #52043 ) ) ;
#66909=CARTESIAN_POINT ( 'NONE',  ( -27.00000000000000000, -1.249999999999999112, 32.75000000000000000 ) ) ;
#66995=EDGE_LOOP ( 'NONE', ( #21830, #75109, #57257, #58444 ) ) ;
#67027=VERTEX_POINT ( 'NONE', #14656 ) ;
#67029=ORIENTED_EDGE ( 'NONE', *, *, #44990, .T. ) ;
#67042=DIRECTION ( 'NONE',  ( -0.000000000000000000, 0.000000000000000000, 1.000000000000000000 ) ) ;
#67184=CARTESIAN_POINT ( 'NONE',  ( -20.00000000000000355, 10.00000000000000711, 13.00000000000000178 ) ) ;
#67238=LINE ( 'NONE', #65882, #83187 ) ;
#67243=LINE ( 'NONE', #30446, #75208 ) ;
#67255=DIRECTION ( 'NONE',  ( 0.000000000000000000, 1.000000000000000000, -2.546383084002652634E-16 ) ) ;
#67273=AXIS2_PLACEMENT_3D ( 'NONE', #13419, #67042, #19737 ) ;
#67370=AXIS2_PLACEMENT_3D ( 'NONE', #64108, #29900, #65880 ) ;
#67441=AXIS2_PLACEMENT_3D ( 'NONE', #10353, #29745, #8590 ) ;
#67477=ORIENTED_EDGE ( 'NONE', *, *, #80257, .F. ) ;
#67503=ORIENTED_EDGE ( 'NONE', *, *, #3518, .T. ) ;
#67511=FILL_AREA_STYLE_COLOUR ( '', #21649 ) ;
#67649=DIRECTION ( 'NONE',  ( 0.000000000000000000, 1.000000000000000000, 8.673617379884034486E-16 ) ) ;
#67678=CIRCLE ( 'NONE', #71976, 8.000000000000000000 ) ;
#67687=VERTEX_POINT ( 'NONE', #28400 ) ;
#67708=LINE ( 'NONE', #6014, #30778 ) ;
#67733=CARTESIAN_POINT ( 'NONE',  ( 23.49999999999998934, -5.499999999999981348, 32.75000000000000000 ) ) ;
#67745=ORIENTED_EDGE ( 'NONE', *, *, #8844, .F. ) ;
#67767=VERTEX_POINT ( 'NONE', #8140 ) ;
#67870=CIRCLE ( 'NONE', #14842, 8.000000000000000000 ) ;
#67901=ORIENTED_EDGE ( 'NONE', *, *, #16116, .T. ) ;
#67945=CARTESIAN_POINT ( 'NONE',  ( 19.00000000000000000, 8.999999999999996447, 23.75000000000000000 ) ) ;
#68008=DIRECTION ( 'NONE',  ( 1.000000000000000000, -0.000000000000000000, -0.000000000000000000 ) ) ;
#68156=ORIENTED_EDGE ( 'NONE', *, *, #27138, .T. ) ;
#68167=CARTESIAN_POINT ( 'NONE',  ( 20.00000000000000355, 10.00000000000000533, 13.00000000000000178 ) ) ;
#68191=CIRCLE ( 'NONE', #66767, 8.000000000000000000 ) ;
#68196=FACE_OUTER_BOUND ( 'NONE', #40387, .T. ) ;
#68210=CARTESIAN_POINT ( 'NONE',  ( -18.23784950573860186, -1.749999999999998668, 30.25000000000000000 ) ) ;
#68221=DIRECTION ( 'NONE',  ( 0.000000000000000000, 0.000000000000000000, -1.000000000000000000 ) ) ;
#68232=CARTESIAN_POINT ( 'NONE',  ( 25.00000000000000355, 9.999999999999971578, 13.00000000000000178 ) ) ;
#68324=EDGE_CURVE ( 'NONE', #36427, #23390, #53931, .T. ) ;
#68363=DIRECTION ( 'NONE',  ( 0.000000000000000000, 0.000000000000000000, -1.000000000000000000 ) ) ;
#68378=EDGE_LOOP ( 'NONE', ( #84331, #63863, #6459, #32308, #31702, #26936 ) ) ;
#68396=EDGE_CURVE ( 'NONE', #43877, #52607, #27306, .T. ) ;
#68470=DIRECTION ( 'NONE',  ( 0.000000000000000000, 0.000000000000000000, -1.000000000000000000 ) ) ;
#68590=EDGE_CURVE ( 'NONE', #81222, #56866, #69754, .T. ) ;
#68607=EDGE_CURVE ( 'NONE', #28603, #8219, #58648, .T. ) ;
#68629=VERTEX_POINT ( 'NONE', #57597 ) ;
#68648=ORIENTED_EDGE ( 'NONE', *, *, #60367, .F. ) ;
#68676=AXIS2_PLACEMENT_3D ( 'NONE', #1230, #76459, #7556 ) ;
#68758=CARTESIAN_POINT ( 'NONE',  ( 24.00000000000000000, -5.499999999999981348, 27.25000000000000000 ) ) ;
#68764=CARTESIAN_POINT ( 'NONE',  ( 27.00000000000000000, 12.75000000000000711, 30.81664701255127881 ) ) ;
#68811=PLANE ( 'NONE',  #82856 ) ;
#68830=DIRECTION ( 'NONE',  ( 0.000000000000000000, 8.673617379884033500E-16, -1.000000000000000000 ) ) ;
#68832=ORIENTED_EDGE ( 'NONE', *, *, #6428, .F. ) ;
#68878=DIRECTION ( 'NONE',  ( 0.000000000000000000, 0.000000000000000000, 1.000000000000000000 ) ) ;
#68913=DIRECTION ( 'NONE',  ( -0.000000000000000000, 1.000000000000000000, -5.102127870520020612E-17 ) ) ;
#68936=EDGE_CURVE ( 'NONE', #5642, #76954, #10009, .T. ) ;
#68963=CARTESIAN_POINT ( 'NONE',  ( -24.00000000000000000, -9.499999999999982236, 27.25000000000000000 ) ) ;
#68964=AXIS2_PLACEMENT_3D ( 'NONE', #63603, #584, #8232 ) ;
#69114=FACE_OUTER_BOUND ( 'NONE', #88109, .T. ) ;
#69115=DIRECTION ( 'NONE',  ( -1.000000000000000000, 0.000000000000000000, 0.000000000000000000 ) ) ;
#69141=ORIENTED_EDGE ( 'NONE', *, *, #74844, .T. ) ;
#69143=ORIENTED_EDGE ( 'NONE', *, *, #74682, .T. ) ;
#69235=LINE ( 'NONE', #22808, #6212 ) ;
#69241=DIRECTION ( 'NONE',  ( 1.000000000000000000, 0.000000000000000000, 0.000000000000000000 ) ) ;
#69299=DIRECTION ( 'NONE',  ( 0.000000000000000000, 0.000000000000000000, -1.000000000000000000 ) ) ;
#69323=CIRCLE ( 'NONE', #41938, 8.000000000000000000 ) ;
#69344=ORIENTED_EDGE ( 'NONE', *, *, #19098, .F. ) ;
#69391=ORIENTED_EDGE ( 'NONE', *, *, #73530, .T. ) ;
#69439=CARTESIAN_POINT ( 'NONE',  ( 19.00000000000000000, -1.250000000000000000, 22.25000000000000000 ) ) ;
#69466=VERTEX_POINT ( 'NONE', #61639 ) ;
#69505=CARTESIAN_POINT ( 'NONE',  ( -19.00000000000000000, 0.7500000000000051070, 32.75000000000000000 ) ) ;
#69519=EDGE_CURVE ( 'NONE', #6010, #3726, #6503, .T. ) ;
#69530=ADVANCED_FACE ( 'NONE', ( #19779 ), #34622, .F. ) ;
#69588=CARTESIAN_POINT ( 'NONE',  ( -19.00000000000000000, -8.999999999999998224, 22.25000000000000000 ) ) ;
#69632=CARTESIAN_POINT ( 'NONE',  ( -18.00000000000000000, 2.999999999999935163, 30.25000000000000000 ) ) ;
#69670=ADVANCED_FACE ( 'NONE', ( #62955 ), #86375, .F. ) ;
#69676=ORIENTED_EDGE ( 'NONE', *, *, #85703, .T. ) ;
#69695=FACE_OUTER_BOUND ( 'NONE', #88128, .T. ) ;
#69754=CIRCLE ( 'NONE', #49567, 8.000000000000000000 ) ;
#69767=DIRECTION ( 'NONE',  ( -1.000000000000000000, -0.000000000000000000, 0.000000000000000000 ) ) ;
#69913=LINE ( 'NONE', #44189, #47535 ) ;
#69979=ORIENTED_EDGE ( 'NONE', *, *, #14033, .T. ) ;
#69991=CYLINDRICAL_SURFACE ( 'NONE', #41574, 4.755951259985877755 ) ;
#70037=ORIENTED_EDGE ( 'NONE', *, *, #85460, .F. ) ;
#70039=CARTESIAN_POINT ( 'NONE',  ( -23.50000000000000000, -8.999999999999996447, 28.86437827766147279 ) ) ;
#70078=FACE_OUTER_BOUND ( 'NONE', #16427, .T. ) ;
#70229=ADVANCED_FACE ( 'NONE', ( #43383 ), #10819, .F. ) ;
#70252=CIRCLE ( 'NONE', #29947, 6.614378277661484340 ) ;
#70291=CARTESIAN_POINT ( 'NONE',  ( -19.00000000000000000, 9.000000000000001776, 2.999999999999999112 ) ) ;
#70334=CARTESIAN_POINT ( 'NONE',  ( 19.00000000000000000, 0.7500000000000051070, 32.75000000000000000 ) ) ;
#70409=DIRECTION ( 'NONE',  ( 0.000000000000000000, 1.000000000000000000, 0.000000000000000000 ) ) ;
#70434=ORIENTED_EDGE ( 'NONE', *, *, #11968, .T. ) ;
#70558=EDGE_CURVE ( 'NONE', #53401, #84701, #54907, .T. ) ;
#70566=ORIENTED_EDGE ( 'NONE', *, *, #39667, .F. ) ;
#70627=ORIENTED_EDGE ( 'NONE', *, *, #33037, .T. ) ;
#70695=ORIENTED_EDGE ( 'NONE', *, *, #51021, .T. ) ;
#70721=ORIENTED_EDGE ( 'NONE', *, *, #34763, .T. ) ;
#70774=EDGE_CURVE ( 'NONE', #4149, #8013, #24663, .T. ) ;
#70803=ADVANCED_FACE ( 'NONE', ( #75083 ), #7508, .F. ) ;
#70831=CARTESIAN_POINT ( 'NONE',  ( -18.23784950573857344, 12.75000000000000711, 30.81664701255125394 ) ) ;
#70848=CARTESIAN_POINT ( 'NONE',  ( 27.00000000000000000, 17.00000000000000000, 2.999999999999999112 ) ) ;
#71003=PLANE ( 'NONE',  #46829 ) ;
#71017=ORIENTED_EDGE ( 'NONE', *, *, #68396, .F. ) ;
#71135=LINE ( 'NONE', #44093, #17389 ) ;
#71247=CARTESIAN_POINT ( 'NONE',  ( -18.07928316857947237, 12.74206001580630598, 30.82086045927834661 ) ) ;
#71255=CARTESIAN_POINT ( 'NONE',  ( -19.00000000000000000, 8.999999999999998224, 23.75000000000000000 ) ) ;
#71314=CARTESIAN_POINT ( 'NONE',  ( -27.00000000000000000, 16.99999999999999289, 23.75000000000000000 ) ) ;
#71315=FACE_OUTER_BOUND ( 'NONE', #47381, .T. ) ;
#71338=ORIENTED_EDGE ( 'NONE', *, *, #73530, .F. ) ;
#71374=ORIENTED_EDGE ( 'NONE', *, *, #81274, .F. ) ;
#71445=EDGE_CURVE ( 'NONE', #14162, #6905, #16760, .T. ) ;
#71522=PRESENTATION_STYLE_ASSIGNMENT (( #44043 ) ) ;
#71544=ORIENTED_EDGE ( 'NONE', *, *, #68590, .F. ) ;
#71636=FACE_OUTER_BOUND ( 'NONE', #14716, .T. ) ;
#71656=ORIENTED_EDGE ( 'NONE', *, *, #65716, .T. ) ;
#71754=VECTOR ( 'NONE', #4993, 1000.000000000000000 ) ;
#71817=CYLINDRICAL_SURFACE ( 'NONE', #53383, 8.000000000000000000 ) ;
#71881=PLANE ( 'NONE',  #11142 ) ;
#71897=CARTESIAN_POINT ( 'NONE',  ( 19.00000000000000000, 8.999999999999996447, 23.75000000000000000 ) ) ;
#71976=AXIS2_PLACEMENT_3D ( 'NONE', #8034, #62513, #1264 ) ;
#71983=ORIENTED_EDGE ( 'NONE', *, *, #55924, .F. ) ;
#72030=ORIENTED_EDGE ( 'NONE', *, *, #56579, .F. ) ;
#72044=PLANE ( 'NONE',  #67441 ) ;
#72080=CIRCLE ( 'NONE', #60628, 5.000000000000000888 ) ;
#72096=VECTOR ( 'NONE', #77597, 1000.000000000000000 ) ;
#72099=VERTEX_POINT ( 'NONE', #22203 ) ;
#72148=DIRECTION ( 'NONE',  ( 9.403954806578300064E-32, -4.336808689942017736E-16, 1.000000000000000000 ) ) ;
#72184=LINE ( 'NONE', #4170, #80123 ) ;
#72262=DIRECTION ( 'NONE',  ( -9.403954806578300064E-32, 4.336808689942017736E-16, 1.000000000000000000 ) ) ;
#72275=CARTESIAN_POINT ( 'NONE',  ( 27.00000000000000000, -1.249999999999999334, 30.25000000000000000 ) ) ;
#72294=ORIENTED_EDGE ( 'NONE', *, *, #2573, .T. ) ;
#72309=CARTESIAN_POINT ( 'NONE',  ( -25.00000000000000355, 9.999999999999971578, 3.000000000000000000 ) ) ;
#72356=DIRECTION ( 'NONE',  ( 0.000000000000000000, -1.000000000000000000, 0.000000000000000000 ) ) ;
#72360=CARTESIAN_POINT ( 'NONE',  ( -27.00000000000000000, 9.000000000000001776, 2.999999999999999556 ) ) ;
#72380=AXIS2_PLACEMENT_3D ( 'NONE', #44878, #72356, #10666 ) ;
#72525=CARTESIAN_POINT ( 'NONE',  ( 27.00000000000000355, -1.749999999999999778, 30.25000000000000000 ) ) ;
#72604=CIRCLE ( 'NONE', #13646, 4.755951259985879531 ) ;
#72783=EDGE_LOOP ( 'NONE', ( #876, #11801, #83243, #5604 ) ) ;
#72866=EDGE_CURVE ( 'NONE', #80750, #19020, #85134, .T. ) ;
#72891=CARTESIAN_POINT ( 'NONE',  ( 23.49999999999998934, 6.011520428872295955E-15, 27.75000000000000355 ) ) ;
#73053=FACE_BOUND ( 'NONE', #86260, .T. ) ;
#73092=LINE ( 'NONE', #32542, #3420 ) ;
#73108=ORIENTED_EDGE ( 'NONE', *, *, #28232, .F. ) ;
#73157=VECTOR ( 'NONE', #54994, 1000.000000000000000 ) ;
#73246=CARTESIAN_POINT ( 'NONE',  ( -17.76215049426127024, 12.75000000000001599, 30.81664701255127881 ) ) ;
#73354=DIRECTION ( 'NONE',  ( 0.000000000000000000, 2.546383084002652634E-16, 1.000000000000000000 ) ) ;
#73362=LINE ( 'NONE', #39147, #52010 ) ;
#73373=( LENGTH_UNIT ( ) NAMED_UNIT ( * ) SI_UNIT ( .MILLI., .METRE. ) );
#73404=CARTESIAN_POINT ( 'NONE',  ( 23.49999999999998934, 1.674711738930281374E-15, 27.25000000000000000 ) ) ;
#73457=CARTESIAN_POINT ( 'NONE',  ( -23.50000000000000000, 8.999999999999996447, 30.36437827766147279 ) ) ;
#73530=EDGE_CURVE ( 'NONE', #84975, #31022, #82715, .T. ) ;
#73534=ORIENTED_EDGE ( 'NONE', *, *, #18680, .T. ) ;
#73537=EDGE_CURVE ( 'NONE', #545, #8013, #61979, .T. ) ;
#73568=ORIENTED_EDGE ( 'NONE', *, *, #31139, .T. ) ;
#73680=EDGE_CURVE ( 'NONE', #57327, #177, #37492, .T. ) ;
#73737=CARTESIAN_POINT ( 'NONE',  ( -23.50000000000000000, -8.999999999999996447, 22.25000000000000000 ) ) ;
#73776=DIRECTION ( 'NONE',  ( 0.000000000000000000, 1.000000000000000000, 0.000000000000000000 ) ) ;
#73791=VECTOR ( 'NONE', #55472, 1000.000000000000000 ) ;
#73822=VERTEX_POINT ( 'NONE', #53681 ) ;
#73909=CIRCLE ( 'NONE', #75391, 8.000000000000000000 ) ;
#73914=VERTEX_POINT ( 'NONE', #7726 ) ;
#73970=ADVANCED_FACE ( 'NONE', ( #9924 ), #58997, .F. ) ;
#74075=CARTESIAN_POINT ( 'NONE',  ( 27.00000000000000000, 9.000000000000001776, 2.172175482962262779E-15 ) ) ;
#74194=AXIS2_PLACEMENT_3D ( 'NONE', #77168, #29001, #36630 ) ;
#74237=CARTESIAN_POINT ( 'NONE',  ( 27.00000000000000000, 0.7500000000000051070, 32.75000000000000000 ) ) ;
#74260=DIRECTION ( 'NONE',  ( 0.000000000000000000, -2.413528314402514090E-16, 1.000000000000000000 ) ) ;
#74305=CARTESIAN_POINT ( 'NONE',  ( 25.00000000000000355, 9.999999999999971578, 13.00000000000000178 ) ) ;
#74342=VECTOR ( 'NONE', #39204, 1000.000000000000000 ) ;
#74580=DIRECTION ( 'NONE',  ( 0.000000000000000000, 0.000000000000000000, 1.000000000000000000 ) ) ;
#74625=LINE ( 'NONE', #29440, #19769 ) ;
#74682=EDGE_CURVE ( 'NONE', #3688, #67767, #81298, .T. ) ;
#74695=VECTOR ( 'NONE', #47915, 1000.000000000000000 ) ;
#74754=PLANE ( 'NONE',  #4613 ) ;
#74844=EDGE_CURVE ( 'NONE', #16480, #65802, #15048, .T. ) ;
#74855=CARTESIAN_POINT ( 'NONE',  ( -27.00000000000000000, -9.000000000000001776, 3.000000000000000444 ) ) ;
#74959=AXIS2_PLACEMENT_3D ( 'NONE', #67945, #83230, #20199 ) ;
#74985=CARTESIAN_POINT ( 'NONE',  ( 19.00000000000000000, -1.249999999999999778, 24.75000000000000000 ) ) ;
#75006=CIRCLE ( 'NONE', #54810, 6.777720855862979121 ) ;
#75083=FACE_OUTER_BOUND ( 'NONE', #75760, .T. ) ;
#75109=ORIENTED_EDGE ( 'NONE', *, *, #48489, .F. ) ;
#75147=VECTOR ( 'NONE', #78613, 1000.000000000000000 ) ;
#75199=EDGE_CURVE ( 'NONE', #545, #50608, #81526, .T. ) ;
#75208=VECTOR ( 'NONE', #26248, 1000.000000000000000 ) ;
#75297=VECTOR ( 'NONE', #38434, 1000.000000000000000 ) ;
#75391=AXIS2_PLACEMENT_3D ( 'NONE', #74985, #20909, #48380 ) ;
#75420=DIRECTION ( 'NONE',  ( 1.000000000000000000, 0.000000000000000000, -0.000000000000000000 ) ) ;
#75423=DIRECTION ( 'NONE',  ( 1.734723475976812518E-16, -1.000000000000000000, 0.000000000000000000 ) ) ;
#75464=ORIENTED_EDGE ( 'NONE', *, *, #58173, .F. ) ;
#75512=DIRECTION ( 'NONE',  ( 0.000000000000000000, -1.000000000000000000, -2.413528314402514090E-16 ) ) ;
#75536=ORIENTED_EDGE ( 'NONE', *, *, #4720, .T. ) ;
#75566=AXIS2_PLACEMENT_3D ( 'NONE', #71897, #25496, #85865 ) ;
#75569=FACE_OUTER_BOUND ( 'NONE', #46450, .T. ) ;
#75707=CARTESIAN_POINT ( 'NONE',  ( -19.99999999999996447, -15.00000000000000533, 3.000000000000000000 ) ) ;
#75731=CARTESIAN_POINT ( 'NONE',  ( 19.00000000000000000, 12.75000000000000711, 23.75000000000000000 ) ) ;
#75743=CARTESIAN_POINT ( 'NONE',  ( -24.00000000000000000, 14.50000000000000533, 1.499999999999997780 ) ) ;
#75760=EDGE_LOOP ( 'NONE', ( #25381, #52672, #35270, #51376 ) ) ;
#75845=CARTESIAN_POINT ( 'NONE',  ( 24.00000000000000000, 9.000000000000024869, 29.25000000000000000 ) ) ;
#75858=CARTESIAN_POINT ( 'NONE',  ( 19.00000000000000000, 8.999999999999998224, 23.75000000000000000 ) ) ;
#75862=EDGE_CURVE ( 'NONE', #56866, #545, #2476, .T. ) ;
#75880=VECTOR ( 'NONE', #48082, 1000.000000000000000 ) ;
#75885=CIRCLE ( 'NONE', #48552, 8.000000000000000000 ) ;
#76016=SPHERICAL_SURFACE ( 'NONE', #74959, 8.000000000000000000 ) ;
#76030=VERTEX_POINT ( 'NONE', #14756 ) ;
#76041=VECTOR ( 'NONE', #43739, 1000.000000000000000 ) ;
#76091=AXIS2_PLACEMENT_3D ( 'NONE', #87157, #25435, #52892 ) ;
#76159=CARTESIAN_POINT ( 'NONE',  ( -20.00000000000000355, 10.00000000000000711, 3.000000000000000000 ) ) ;
#76174=VERTEX_POINT ( 'NONE', #12427 ) ;
#76195=CIRCLE ( 'NONE', #48864, 5.000000000000000888 ) ;
#76270=ORIENTED_EDGE ( 'NONE', *, *, #21917, .T. ) ;
#76342=FACE_OUTER_BOUND ( 'NONE', #2506, .T. ) ;
#76425=DIRECTION ( 'NONE',  ( -0.000000000000000000, 2.413528314402514090E-16, -1.000000000000000000 ) ) ;
#76459=DIRECTION ( 'NONE',  ( 0.000000000000000000, 0.000000000000000000, 1.000000000000000000 ) ) ;
#76460=LINE ( 'NONE', #40901, #49479 ) ;
#76465=EDGE_LOOP ( 'NONE', ( #30230, #1117, #32923, #42290, #63433 ) ) ;
#76515=ORIENTED_EDGE ( 'NONE', *, *, #69519, .T. ) ;
#76542=CARTESIAN_POINT ( 'NONE',  ( -19.00000000000000000, -13.25000000000000533, 29.02772085586297024 ) ) ;
#76662=EDGE_CURVE ( 'NONE', #78849, #5642, #31348, .T. ) ;
#76688=DIRECTION ( 'NONE',  ( 0.000000000000000000, 1.000000000000000000, 0.000000000000000000 ) ) ;
#76730=DIRECTION ( 'NONE',  ( -0.000000000000000000, 1.000000000000000000, -0.000000000000000000 ) ) ;
#76759=EDGE_CURVE ( 'NONE', #2885, #81222, #58952, .T. ) ;
#76954=VERTEX_POINT ( 'NONE', #7127 ) ;
#76989=DIRECTION ( 'NONE',  ( 0.000000000000000000, -1.000000000000000000, -2.413528314402514090E-16 ) ) ;
#77030=VERTEX_POINT ( 'NONE', #50306 ) ;
#77089=EDGE_LOOP ( 'NONE', ( #44653, #73534, #43600, #70721, #27957, #9143 ) ) ;
#77134=AXIS2_PLACEMENT_3D ( 'NONE', #58543, #85151, #52237 ) ;
#77162=ORIENTED_EDGE ( 'NONE', *, *, #37911, .T. ) ;
#77168=CARTESIAN_POINT ( 'NONE',  ( 27.00000000000000000, 0.7500000000000051070, 32.75000000000000000 ) ) ;
#77195=VECTOR ( 'NONE', #17817, 1000.000000000000000 ) ;
#77196=DIRECTION ( 'NONE',  ( -0.000000000000000000, -5.102127870520021228E-17, -1.000000000000000000 ) ) ;
#77232=CARTESIAN_POINT ( 'NONE',  ( -19.00000000000000000, -1.749999999999991118, 22.25000000000000000 ) ) ;
#77270=CARTESIAN_POINT ( 'NONE',  ( 19.00000000000000355, -13.24999999999999822, 29.02772085586297734 ) ) ;
#77293=ORIENTED_EDGE ( 'NONE', *, *, #56069, .T. ) ;
#77520=CARTESIAN_POINT ( 'NONE',  ( 23.49999999999998579, -1.749999999999999556, 32.75000000000000000 ) ) ;
#77570=CYLINDRICAL_SURFACE ( 'NONE', #43855, 8.000000000000000000 ) ;
#77574=ADVANCED_FACE ( 'NONE', ( #20436 ), #6483, .T. ) ;
#77597=DIRECTION ( 'NONE',  ( -1.000000000000000000, -0.000000000000000000, -0.000000000000000000 ) ) ;
#77708=AXIS2_PLACEMENT_3D ( 'NONE', #18018, #31066, #77932 ) ;
#77763=CARTESIAN_POINT ( 'NONE',  ( -24.00000000000000000, 9.000000000000024869, 29.25000000000000000 ) ) ;
#77932=DIRECTION ( 'NONE',  ( 1.000000000000000000, -5.997714145664496128E-17, 0.000000000000000000 ) ) ;
#78005=CARTESIAN_POINT ( 'NONE',  ( 19.00000000000000000, -1.749999999999998890, 30.25000000000000000 ) ) ;
#78062=ORIENTED_EDGE ( 'NONE', *, *, #22131, .T. ) ;
#78112=VERTEX_POINT ( 'NONE', #75707 ) ;
#78133=VECTOR ( 'NONE', #14851, 1000.000000000000000 ) ;
#78144=ORIENTED_EDGE ( 'NONE', *, *, #12529, .T. ) ;
#78170=CARTESIAN_POINT ( 'NONE',  ( -24.00000000000000000, -9.499999999999982236, 27.25000000000000000 ) ) ;
#78277=SURFACE_STYLE_FILL_AREA ( #2179 ) ;
#78318=DIRECTION ( 'NONE',  ( -0.000000000000000000, -0.000000000000000000, -1.000000000000000000 ) ) ;
#78339=CARTESIAN_POINT ( 'NONE',  ( 24.00000000000000000, 9.000000000000024869, 29.25000000000000000 ) ) ;
#78453=VECTOR ( 'NONE', #13855, 1000.000000000000000 ) ;
#78493=LINE ( 'NONE', #16794, #34970 ) ;
#78541=EDGE_CURVE ( 'NONE', #72099, #16365, #45700, .T. ) ;
#78562=ADVANCED_FACE ( 'NONE', ( #31755 ), #59657, .T. ) ;
#78582=EDGE_CURVE ( 'NONE', #69466, #6010, #88936, .T. ) ;
#78613=DIRECTION ( 'NONE',  ( 1.000000000000000000, -0.000000000000000000, -0.000000000000000000 ) ) ;
#78620=ORIENTED_EDGE ( 'NONE', *, *, #58823, .F. ) ;
#78720=DIRECTION ( 'NONE',  ( -0.000000000000000000, 1.000000000000000000, -0.000000000000000000 ) ) ;
#78757=ORIENTED_EDGE ( 'NONE', *, *, #75199, .T. ) ;
#78849=VERTEX_POINT ( 'NONE', #68232 ) ;
#78945=ADVANCED_FACE ( 'NONE', ( #71315 ), #69991, .T. ) ;
#79080=ORIENTED_EDGE ( 'NONE', *, *, #21087, .T. ) ;
#79136=DIRECTION ( 'NONE',  ( -0.000000000000000000, 0.000000000000000000, 1.000000000000000000 ) ) ;
#79175=CARTESIAN_POINT ( 'NONE',  ( 23.49999999999998579, -1.749999999999999778, 28.86437827766148345 ) ) ;
#79192=STYLED_ITEM ( 'NONE', ( #7579 ), #38570 ) ;
#79194=EDGE_CURVE ( 'NONE', #8219, #1369, #42870, .T. ) ;
#79212=ORIENTED_EDGE ( 'NONE', *, *, #16138, .T. ) ;
#79335=DIRECTION ( 'NONE',  ( 0.000000000000000000, 1.000000000000000000, -0.000000000000000000 ) ) ;
#79337=VECTOR ( 'NONE', #19307, 1000.000000000000000 ) ;
#79377=DIRECTION ( 'NONE',  ( -0.000000000000000000, -5.102127870520021228E-17, -1.000000000000000000 ) ) ;
#79425=FACE_BOUND ( 'NONE', #50660, .T. ) ;
#79431=VERTEX_POINT ( 'NONE', #40002 ) ;
#79493=ORIENTED_EDGE ( 'NONE', *, *, #22887, .T. ) ;
#79499=CARTESIAN_POINT ( 'NONE',  ( 19.99999999999997158, -14.99999999999999467, 13.00000000000000178 ) ) ;
#79516=CARTESIAN_POINT ( 'NONE',  ( -17.76215049426128445, -1.749999999999992228, 32.75000000000000000 ) ) ;
#79532=DIRECTION ( 'NONE',  ( 0.000000000000000000, 1.000000000000000000, 0.000000000000000000 ) ) ;
#79546=CARTESIAN_POINT ( 'NONE',  ( 24.00000000000000000, 5.000000000000023093, 29.24999999999999645 ) ) ;
#79547=VERTEX_POINT ( 'NONE', #43961 ) ;
#79573=VERTEX_POINT ( 'NONE', #50262 ) ;
#79587=CARTESIAN_POINT ( 'NONE',  ( 24.00000000000000000, -9.499999999999982236, 27.74999999999999645 ) ) ;
#79605=CARTESIAN_POINT ( 'NONE',  ( -19.00000000000000000, -1.249999999999999112, 32.75000000000000000 ) ) ;
#79644=EDGE_CURVE ( 'NONE', #26806, #11121, #63790, .T. ) ;
#79822=FACE_OUTER_BOUND ( 'NONE', #6949, .T. ) ;
#79853=AXIS2_PLACEMENT_3D ( 'NONE', #20226, #35509, #82819 ) ;
#79929=CARTESIAN_POINT ( 'NONE',  ( -18.23784950573860186, -1.749999999999998446, 32.75000000000000000 ) ) ;
#79945=AXIS2_PLACEMENT_3D ( 'NONE', #87424, #19391, #25705 ) ;
#79969=LINE ( 'NONE', #60577, #83922 ) ;
#80003=CARTESIAN_POINT ( 'NONE',  ( -18.00000000000001421, 17.49999999999802824, 13.00000000000000178 ) ) ;
#80004=CARTESIAN_POINT ( 'NONE',  ( -3.148799926473854489E-16, -1.749999999999995781, 28.00000000000000000 ) ) ;
#80064=( LENGTH_UNIT ( ) NAMED_UNIT ( * ) SI_UNIT ( .MILLI., .METRE. ) );
#80065=VECTOR ( 'NONE', #67649, 1000.000000000000000 ) ;
#80123=VECTOR ( 'NONE', #23990, 1000.000000000000000 ) ;
#80193=DIRECTION ( 'NONE',  ( 1.000000000000000000, -0.000000000000000000, -0.000000000000000000 ) ) ;
#80257=EDGE_CURVE ( 'NONE', #65802, #28603, #22915, .T. ) ;
#80311=DIRECTION ( 'NONE',  ( 0.000000000000000000, 0.000000000000000000, 1.000000000000000000 ) ) ;
#80332=LINE ( 'NONE', #18623, #43667 ) ;
#80430=EDGE_CURVE ( 'NONE', #77030, #73914, #33794, .T. ) ;
#80432=CLOSED_SHELL ( 'NONE', ( #61668, #87292, #6795, #45823, #9245, #70229, #26409, #87206, #33249, #70803, #83177, #47872, #65749, #54554, #33636, #22224, #84412, #78562, #25785, #34429, #59791, #56895, #85622, #19625, #82571, #45438, #45830, #47751, #78945, #62877, #41635, #18905, #77574, #63827, #45071, #717, #43299, #19144, #83954, #54870, #65660, #60433, #73970, #52206, #31287, #31608, #8746, #43171, #32757, #13181, #6323, #35896, #64539, #53184, #21691, #14820, #69530, #35992, #15326, #53314, #21406, #63175, #5342, #69670, #49723, #65060 ) ) ;
#80452=ORIENTED_EDGE ( 'NONE', *, *, #8750, .T. ) ;
#80523=EDGE_LOOP ( 'NONE', ( #84626, #40909, #2785, #39192 ) ) ;
#80572=DIRECTION ( 'NONE',  ( 0.000000000000000000, -1.000000000000000000, 4.336808689942018722E-16 ) ) ;
#80595=ORIENTED_EDGE ( 'NONE', *, *, #38642, .F. ) ;
#80606=FACE_OUTER_BOUND ( 'NONE', #4886, .T. ) ;
#80635=( GEOMETRIC_REPRESENTATION_CONTEXT ( 3 ) GLOBAL_UNCERTAINTY_ASSIGNED_CONTEXT ( ( #16731 ) ) GLOBAL_UNIT_ASSIGNED_CONTEXT ( ( #73373, #25629, #5363 ) ) REPRESENTATION_CONTEXT ( 'NONE', 'WORKASPACE' ) );
#80639=CARTESIAN_POINT ( 'NONE',  ( -27.00000000000000000, -8.999999999999994671, 30.24999999999999645 ) ) ;
#80645=CARTESIAN_POINT ( 'NONE',  ( -23.50000000000000000, -1.749999999999992006, 28.00000000000000000 ) ) ;
#80654=ORIENTED_EDGE ( 'NONE', *, *, #82394, .T. ) ;
#80670=EDGE_CURVE ( 'NONE', #50608, #72099, #17511, .T. ) ;
#80699=DIRECTION ( 'NONE',  ( 1.000000000000000000, -0.000000000000000000, -0.000000000000000000 ) ) ;
#80750=VERTEX_POINT ( 'NONE', #48856 ) ;
#80760=PLANE ( 'NONE',  #42946 ) ;
#80770=EDGE_LOOP ( 'NONE', ( #55176, #82987, #49186, #18122 ) ) ;
#80935=ORIENTED_EDGE ( 'NONE', *, *, #26174, .F. ) ;
#80947=CARTESIAN_POINT ( 'NONE',  ( -24.00000000000000000, -5.499999999999981348, 27.75000000000000000 ) ) ;
#81019=LINE ( 'NONE', #18863, #79337 ) ;
#81076=DIRECTION ( 'NONE',  ( 0.000000000000000000, -1.000000000000000000, -1.084202172485503448E-16 ) ) ;
#81222=VERTEX_POINT ( 'NONE', #85210 ) ;
#81251=ORIENTED_EDGE ( 'NONE', *, *, #79194, .T. ) ;
#81274=EDGE_CURVE ( 'NONE', #67767, #1369, #69913, .T. ) ;
#81298=LINE ( 'NONE', #79516, #77195 ) ;
#81327=EDGE_LOOP ( 'NONE', ( #34868, #21533, #78620, #42529 ) ) ;
#81372=ORIENTED_EDGE ( 'NONE', *, *, #33771, .T. ) ;
#81392=EDGE_CURVE ( 'NONE', #85470, #50608, #34563, .T. ) ;
#81407=ORIENTED_EDGE ( 'NONE', *, *, #88503, .F. ) ;
#81453=PLANE ( 'NONE',  #67273 ) ;
#81526=CIRCLE ( 'NONE', #84413, 6.614378277661474570 ) ;
#81553=VECTOR ( 'NONE', #68008, 1000.000000000000000 ) ;
#81578=ORIENTED_EDGE ( 'NONE', *, *, #87020, .F. ) ;
#81696=LINE ( 'NONE', #67733, #65718 ) ;
#81713=AXIS2_PLACEMENT_3D ( 'NONE', #29400, #63607, #20849 ) ;
#81793=ORIENTED_EDGE ( 'NONE', *, *, #45616, .T. ) ;
#81807=AXIS2_PLACEMENT_3D ( 'NONE', #46784, #66617, #5357 ) ;
#81842=CARTESIAN_POINT ( 'NONE',  ( 27.00000000000000000, 16.99999999999999289, 31.75000000000000000 ) ) ;
#81950=FACE_OUTER_BOUND ( 'NONE', #45193, .T. ) ;
#81951=DIRECTION ( 'NONE',  ( -1.000000000000000000, -0.000000000000000000, -0.000000000000000000 ) ) ;
#81965=LINE ( 'NONE', #13488, #63792 ) ;
#81984=LINE ( 'NONE', #62135, #27180 ) ;
#82054=LINE ( 'NONE', #13582, #80065 ) ;
#82079=DIRECTION ( 'NONE',  ( 0.000000000000000000, 0.000000000000000000, -1.000000000000000000 ) ) ;
#82089=AXIS2_PLACEMENT_3D ( 'NONE', #77232, #15542, #43010 ) ;
#82133=FACE_OUTER_BOUND ( 'NONE', #46684, .T. ) ;
#82359=( LENGTH_UNIT ( ) NAMED_UNIT ( * ) SI_UNIT ( .MILLI., .METRE. ) );
#82394=EDGE_CURVE ( 'NONE', #41015, #43004, #71135, .T. ) ;
#82439=CIRCLE ( 'NONE', #4766, 8.000000000000000000 ) ;
#82509=AXIS2_PLACEMENT_3D ( 'NONE', #39778, #19051, #52822 ) ;
#82521=ORIENTED_EDGE ( 'NONE', *, *, #34020, .F. ) ;
#82571=ADVANCED_FACE ( 'NONE', ( #55740 ), #76016, .T. ) ;
#82584=CYLINDRICAL_SURFACE ( 'NONE', #72380, 8.000000000000000000 ) ;
#82588=ORIENTED_EDGE ( 'NONE', *, *, #68607, .F. ) ;
#82658=AXIS2_PLACEMENT_3D ( 'NONE', #59535, #6808, #61296 ) ;
#82678=DIRECTION ( 'NONE',  ( 0.000000000000000000, 8.673617379884028076E-17, 1.000000000000000000 ) ) ;
#82715=LINE ( 'NONE', #2374, #18127 ) ;
#82720=DIRECTION ( 'NONE',  ( -1.000000000000000000, 0.000000000000000000, 0.000000000000000000 ) ) ;
#82742=FACE_OUTER_BOUND ( 'NONE', #82791, .T. ) ;
#82762=EDGE_LOOP ( 'NONE', ( #659, #86392, #44063, #46782 ) ) ;
#82791=EDGE_LOOP ( 'NONE', ( #85355, #62566, #54260, #3976, #33093, #17614, #25546, #78062 ) ) ;
#82819=DIRECTION ( 'NONE',  ( 0.000000000000000000, -1.000000000000000000, -4.336808689942017736E-16 ) ) ;
#82856=AXIS2_PLACEMENT_3D ( 'NONE', #35468, #13422, #34585 ) ;
#82872=VECTOR ( 'NONE', #81951, 1000.000000000000000 ) ;
#82956=LINE ( 'NONE', #976, #73791 ) ;
#82987=ORIENTED_EDGE ( 'NONE', *, *, #53801, .T. ) ;
#83081=DIRECTION ( 'NONE',  ( 1.000000000000000000, -1.681660752236433198E-16, 0.000000000000000000 ) ) ;
#83177=ADVANCED_FACE ( 'NONE', ( #44214 ), #44660, .F. ) ;
#83182=ORIENTED_EDGE ( 'NONE', *, *, #7435, .T. ) ;
#83187=VECTOR ( 'NONE', #45171, 1000.000000000000000 ) ;
#83225=CARTESIAN_POINT ( 'NONE',  ( -19.99999999999996803, 15.00000000000000711, 13.00000000000000178 ) ) ;
#83229=DIRECTION ( 'NONE',  ( 0.000000000000000000, 0.000000000000000000, -1.000000000000000000 ) ) ;
#83230=DIRECTION ( 'NONE',  ( 1.000000000000000000, 0.000000000000000000, -0.000000000000000000 ) ) ;
#83243=ORIENTED_EDGE ( 'NONE', *, *, #64166, .T. ) ;
#83306=FACE_OUTER_BOUND ( 'NONE', #82762, .T. ) ;
#83331=EDGE_LOOP ( 'NONE', ( #753, #24955, #125, #80595 ) ) ;
#83448=AXIS2_PLACEMENT_3D ( 'NONE', #62763, #83959, #35307 ) ;
#83500=DIRECTION ( 'NONE',  ( 0.000000000000000000, -1.000000000000000000, 0.000000000000000000 ) ) ;
#83507=AXIS2_PLACEMENT_3D ( 'NONE', #39698, #79335, #85649 ) ;
#83746=ORIENTED_EDGE ( 'NONE', *, *, #50706, .T. ) ;
#83751=PLANE ( 'NONE',  #58011 ) ;
#83808=CARTESIAN_POINT ( 'NONE',  ( -1.105886215935217836E-14, 12.75000000000002665, 32.75000000000000000 ) ) ;
#83817=ORIENTED_EDGE ( 'NONE', *, *, #48489, .T. ) ;
#83871=ORIENTED_EDGE ( 'NONE', *, *, #58219, .F. ) ;
#83909=CARTESIAN_POINT ( 'NONE',  ( 19.00000000000000000, 0.7500000000000052180, 31.75000000000000000 ) ) ;
#83922=VECTOR ( 'NONE', #79532, 1000.000000000000000 ) ;
#83954=ADVANCED_FACE ( 'NONE', ( #17521 ), #65247, .F. ) ;
#83959=DIRECTION ( 'NONE',  ( 0.000000000000000000, 0.000000000000000000, 1.000000000000000000 ) ) ;
#84010=PLANE ( 'NONE',  #64957 ) ;
#84015=CARTESIAN_POINT ( 'NONE',  ( 23.49999999999998579, 1.250000000000000666, 30.36437827766148345 ) ) ;
#84056=DIRECTION ( 'NONE',  ( 0.000000000000000000, -0.000000000000000000, 1.000000000000000000 ) ) ;
#84085=LINE ( 'NONE', #21475, #44895 ) ;
#84135=DIRECTION ( 'NONE',  ( -1.000000000000000000, -0.000000000000000000, 0.000000000000000000 ) ) ;
#84203=LINE ( 'NONE', #7648, #40676 ) ;
#84204=CARTESIAN_POINT ( 'NONE',  ( 19.00000000000000000, 9.000000000000001776, 2.172175482962262779E-15 ) ) ;
#84256=EDGE_LOOP ( 'NONE', ( #53675, #20286, #32225, #77293 ) ) ;
#84301=CARTESIAN_POINT ( 'NONE',  ( -25.00000000000000355, 9.999999999999971578, 13.00000000000000178 ) ) ;
#84331=ORIENTED_EDGE ( 'NONE', *, *, #68607, .T. ) ;
#84412=ADVANCED_FACE ( 'NONE', ( #47089 ), #61053, .T. ) ;
#84413=AXIS2_PLACEMENT_3D ( 'NONE', #26403, #25952, #60173 ) ;
#84428=LINE ( 'NONE', #64122, #45601 ) ;
#84439=VECTOR ( 'NONE', #49035, 1000.000000000000000 ) ;
#84626=ORIENTED_EDGE ( 'NONE', *, *, #31139, .F. ) ;
#84638=EDGE_CURVE ( 'NONE', #36427, #63016, #26009, .T. ) ;
#84639=LINE ( 'NONE', #58459, #46708 ) ;
#84676=LINE ( 'NONE', #30157, #53021 ) ;
#84701=VERTEX_POINT ( 'NONE', #11440 ) ;
#84759=ORIENTED_EDGE ( 'NONE', *, *, #79644, .T. ) ;
#84776=DIRECTION ( 'NONE',  ( -0.000000000000000000, 1.000000000000000000, 1.084202172485503448E-16 ) ) ;
#84907=FACE_OUTER_BOUND ( 'NONE', #45727, .T. ) ;
#84957=EDGE_CURVE ( 'NONE', #32798, #46479, #42469, .T. ) ;
#84975=VERTEX_POINT ( 'NONE', #4003 ) ;
#85069=VECTOR ( 'NONE', #34659, 1000.000000000000000 ) ;
#85092=VECTOR ( 'NONE', #45770, 1000.000000000000000 ) ;
#85134=LINE ( 'NONE', #4025, #16823 ) ;
#85151=DIRECTION ( 'NONE',  ( -0.000000000000000000, -0.000000000000000000, -1.000000000000000000 ) ) ;
#85173=VECTOR ( 'NONE', #87715, 1000.000000000000000 ) ;
#85181=ORIENTED_EDGE ( 'NONE', *, *, #74682, .F. ) ;
#85187=ORIENTED_EDGE ( 'NONE', *, *, #3601, .T. ) ;
#85210=CARTESIAN_POINT ( 'NONE',  ( -19.00000000000000000, 16.99999999999999645, 23.75000000000000355 ) ) ;
#85213=LINE ( 'NONE', #59057, #43711 ) ;
#85355=ORIENTED_EDGE ( 'NONE', *, *, #32193, .F. ) ;
#85389=ORIENTED_EDGE ( 'NONE', *, *, #23773, .F. ) ;
#85460=EDGE_CURVE ( 'NONE', #4430, #36427, #32709, .T. ) ;
#85470=VERTEX_POINT ( 'NONE', #19643 ) ;
#85607=AXIS2_PLACEMENT_3D ( 'NONE', #84204, #56270, #76989 ) ;
#85620=ORIENTED_EDGE ( 'NONE', *, *, #55492, .T. ) ;
#85622=ADVANCED_FACE ( 'NONE', ( #84907 ), #71817, .T. ) ;
#85627=VECTOR ( 'NONE', #30288, 1000.000000000000000 ) ;
#85635=EDGE_CURVE ( 'NONE', #57828, #79573, #64884, .T. ) ;
#85649=DIRECTION ( 'NONE',  ( 0.000000000000000000, 0.000000000000000000, 1.000000000000000000 ) ) ;
#85703=EDGE_CURVE ( 'NONE', #18166, #423, #52879, .T. ) ;
#85865=DIRECTION ( 'NONE',  ( -8.673617379884035472E-16, 0.000000000000000000, 1.000000000000000000 ) ) ;
#85984=EDGE_CURVE ( 'NONE', #58506, #2885, #10912, .T. ) ;
#86056=VECTOR ( 'NONE', #52921, 1000.000000000000000 ) ;
#86101=DIRECTION ( 'NONE',  ( -0.000000000000000000, -8.673617379884035472E-17, -1.000000000000000000 ) ) ;
#86206=AXIS2_PLACEMENT_3D ( 'NONE', #41811, #84135, #89125 ) ;
#86248=DIRECTION ( 'NONE',  ( 0.000000000000000000, 0.000000000000000000, 1.000000000000000000 ) ) ;
#86260=EDGE_LOOP ( 'NONE', ( #36601, #39724, #40098, #75536 ) ) ;
#86315=ORIENTED_EDGE ( 'NONE', *, *, #22029, .T. ) ;
#86338=LINE ( 'NONE', #52073, #11416 ) ;
#86375=PLANE ( 'NONE',  #12341 ) ;
#86392=ORIENTED_EDGE ( 'NONE', *, *, #45616, .F. ) ;
#86435=ORIENTED_EDGE ( 'NONE', *, *, #30197, .F. ) ;
#86445=DIRECTION ( 'NONE',  ( 0.000000000000000000, -5.102127870520020612E-17, -1.000000000000000000 ) ) ;
#86503=PLANE ( 'NONE',  #29350 ) ;
#86542=ORIENTED_EDGE ( 'NONE', *, *, #66336, .F. ) ;
#86557=CARTESIAN_POINT ( 'NONE',  ( -18.00000000000000000, 2.999999999999934719, 28.00000000000000000 ) ) ;
#86597=ORIENTED_EDGE ( 'NONE', *, *, #15624, .F. ) ;
#86633=VECTOR ( 'NONE', #16578, 1000.000000000000000 ) ;
#86767=ORIENTED_EDGE ( 'NONE', *, *, #65716, .F. ) ;
#86794=LINE ( 'NONE', #13662, #523 ) ;
#86877=EDGE_LOOP ( 'NONE', ( #8863, #27923, #80452, #84759 ) ) ;
#86987=LINE ( 'NONE', #53158, #71754 ) ;
#86991=ORIENTED_EDGE ( 'NONE', *, *, #4720, .F. ) ;
#87020=EDGE_CURVE ( 'NONE', #8013, #45114, #54540, .T. ) ;
#87152=ORIENTED_EDGE ( 'NONE', *, *, #85703, .F. ) ;
#87157=CARTESIAN_POINT ( 'NONE',  ( -19.00000000000000000, -8.999999999999996447, 22.25000000000000000 ) ) ;
#87202=CARTESIAN_POINT ( 'NONE',  ( 27.00000000000000000, -17.00000000000000000, 2.999999999999999112 ) ) ;
#87206=ADVANCED_FACE ( 'NONE', ( #3136 ), #72044, .F. ) ;
#87269=LINE ( 'NONE', #39964, #47491 ) ;
#87292=ADVANCED_FACE ( 'NONE', ( #38269, #80606, #19336 ), #66173, .F. ) ;
#87333=CARTESIAN_POINT ( 'NONE',  ( -19.00000000000000000, -8.999999999999996447, 22.25000000000000000 ) ) ;
#87342=FACE_OUTER_BOUND ( 'NONE', #9065, .T. ) ;
#87377=LINE ( 'NONE', #73404, #36156 ) ;
#87424=CARTESIAN_POINT ( 'NONE',  ( 24.00000000000000000, 0.000000000000000000, 0.000000000000000000 ) ) ;
#87499=DIRECTION ( 'NONE',  ( -0.000000000000000000, -1.000000000000000000, 8.673617379884028076E-17 ) ) ;
#87547=DIRECTION ( 'NONE',  ( 0.000000000000000000, 1.000000000000000000, 0.000000000000000000 ) ) ;
#87661=AXIS2_PLACEMENT_3D ( 'NONE', #15329, #36482, #14890 ) ;
#87698=VERTEX_POINT ( 'NONE', #48017 ) ;
#87715=DIRECTION ( 'NONE',  ( 0.000000000000000000, -1.000000000000000000, 0.000000000000000000 ) ) ;
#87746=EDGE_CURVE ( 'NONE', #58097, #52311, #41720, .T. ) ;
#87747=CARTESIAN_POINT ( 'NONE',  ( 26.99999999999999645, 12.75000000000004974, 30.81664701255125394 ) ) ;
#87845=VECTOR ( 'NONE', #10253, 1000.000000000000000 ) ;
#87852=DIRECTION ( 'NONE',  ( 0.000000000000000000, 1.084202172485504434E-16, -1.000000000000000000 ) ) ;
#87882=PLANE ( 'NONE',  #79945 ) ;
#87883=VERTEX_POINT ( 'NONE', #77270 ) ;
#87965=EDGE_LOOP ( 'NONE', ( #10742, #70566, #71656, #31476 ) ) ;
#88071=AXIS2_PLACEMENT_3D ( 'NONE', #75845, #83500, #21786 ) ;
#88109=EDGE_LOOP ( 'NONE', ( #45381, #49268, #19122, #439, #8098 ) ) ;
#88128=EDGE_LOOP ( 'NONE', ( #32921, #6589, #79212, #83817 ) ) ;
#88176=VERTEX_POINT ( 'NONE', #55123 ) ;
#88190=ORIENTED_EDGE ( 'NONE', *, *, #78541, .T. ) ;
#88193=DIRECTION ( 'NONE',  ( 0.000000000000000000, 0.000000000000000000, 1.000000000000000000 ) ) ;
#88238=AXIS2_PLACEMENT_3D ( 'NONE', #61457, #54256, #83081 ) ;
#88334=FACE_OUTER_BOUND ( 'NONE', #36310, .T. ) ;
#88340=EDGE_CURVE ( 'NONE', #64684, #61438, #47366, .T. ) ;
#88476=DIRECTION ( 'NONE',  ( 0.000000000000000000, 1.000000000000000000, 0.000000000000000000 ) ) ;
#88503=EDGE_CURVE ( 'NONE', #32798, #1675, #5952, .T. ) ;
#88514=FACE_OUTER_BOUND ( 'NONE', #52032, .T. ) ;
#88613=PLANE ( 'NONE',  #13920 ) ;
#88718=PLANE ( 'NONE',  #18320 ) ;
#88764=DIRECTION ( 'NONE',  ( -1.000000000000000000, -0.000000000000000000, -0.000000000000000000 ) ) ;
#88830=VERTEX_POINT ( 'NONE', #68758 ) ;
#88839=VERTEX_POINT ( 'NONE', #48926 ) ;
#88936=LINE ( 'NONE', #74075, #74695 ) ;
#88945=FACE_OUTER_BOUND ( 'NONE', #86877, .T. ) ;
#88983=EDGE_LOOP ( 'NONE', ( #33391, #30250, #3878, #21024 ) ) ;
#89125=DIRECTION ( 'NONE',  ( 0.000000000000000000, 1.835858764360062270E-15, -1.000000000000000000 ) ) ;
ENDSEC;
END-ISO-10303-21;
